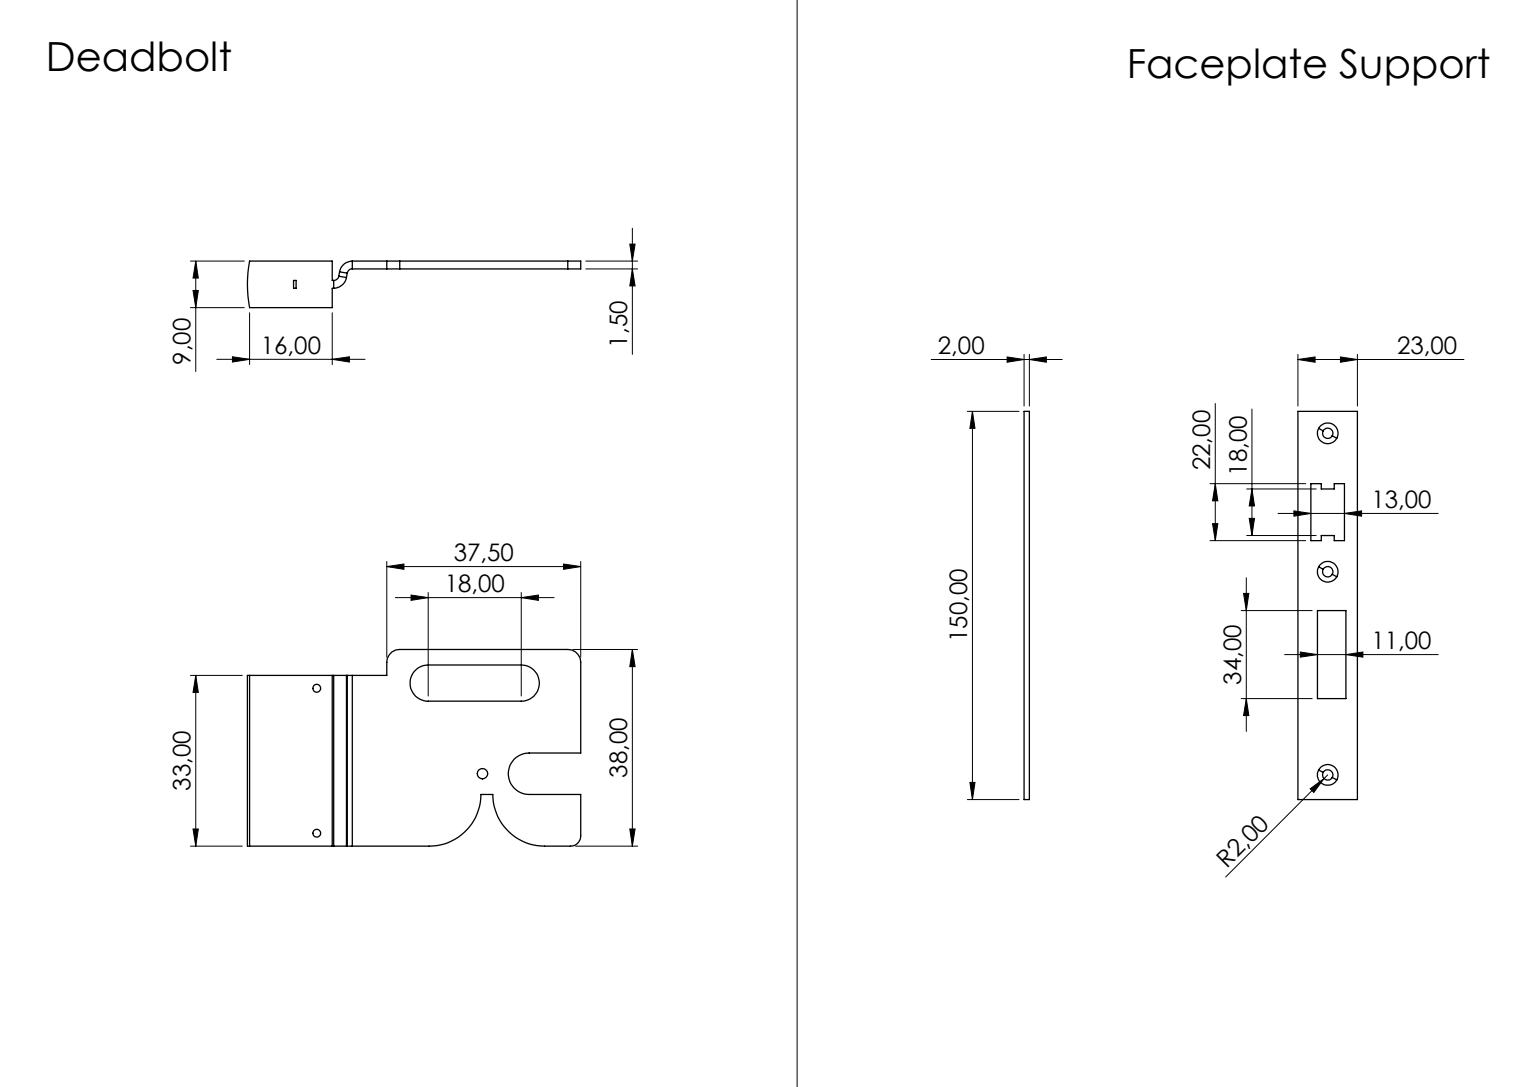
ISO-10303-21;
HEADER;
FILE_DESCRIPTION (('STEP AP214'),
    '1' );
FILE_NAME ('Deadbolt.step',
    '2026-10-06T13:23:30',
    ( '' ),
    ( '' ),
    'SwSTEP 2.0',
    'SolidWorks 2020',
    '' );
FILE_SCHEMA (( 'AUTOMOTIVE_DESIGN' ));
ENDSEC;

DATA;
#1=VERTEX_POINT ( 'NONE', #187 ) ;
#18=ORIENTED_EDGE ( 'NONE', *, *, #14112, .F. ) ;
#27=EDGE_LOOP ( 'NONE', ( #14113, #8328, #12180, #9090 ) ) ;
#42=DIRECTION ( 'NONE',  ( 0.000000000000000000, 1.000000000000000000, 0.000000000000000000 ) ) ;
#43=DIRECTION ( 'NONE',  ( 0.000000000000000000, 1.000000000000000000, 0.000000000000000000 ) ) ;
#46=CARTESIAN_POINT ( 'NONE',  ( -26.35824191589999899, -34.50000000000000000, -150.0657682190000060 ) ) ;
#49=DIRECTION ( 'NONE',  ( -2.507771768020000122E-12, -0.000000000000000000, 1.000000000000000000 ) ) ;
#77=AXIS2_PLACEMENT_3D ( 'NONE', #19282, #2992, #15716 ) ;
#116=MECHANICAL_DESIGN_GEOMETRIC_PRESENTATION_REPRESENTATION('',(#11103),#3517);
#123=CARTESIAN_POINT ( 'NONE',  ( 10.38320006080000013, -24.50000000000000000, -148.5552959529999839 ) ) ;
#126=DIRECTION ( 'NONE',  ( 0.000000000000000000, 0.000000000000000000, 1.000000000000000000 ) ) ;
#136=LINE ( 'NONE', #21434, #17431 ) ;
#139=CARTESIAN_POINT ( 'NONE',  ( -26.35824191589999899, -34.50000000000000000, -141.0657682190000060 ) ) ;
#140=CARTESIAN_POINT ( 'NONE',  ( -18.07392865170000107, -1.500000000000000000, -147.3157682190000060 ) ) ;
#154=VERTEX_POINT ( 'NONE', #4337 ) ;
#161=AXIS2_PLACEMENT_3D ( 'NONE', #17240, #17123, #840 ) ;
#163=DIRECTION ( 'NONE',  ( -2.808280234689999718E-18, 1.000000000000000000, 1.592654863519999645E-17 ) ) ;
#172=ADVANCED_FACE ( 'NONE', ( #21960 ), #4222, .F. ) ;
#175=CARTESIAN_POINT ( 'NONE',  ( -7.816799939239999162, -1.500000000000000000, -148.5552959529999839 ) ) ;
#176=DIRECTION ( 'NONE',  ( 2.507771768019999718E-12, 1.592654864069999939E-17, -1.000000000000000000 ) ) ;
#187=CARTESIAN_POINT ( 'NONE',  ( -20.60824191591068555, -32.00000000000000000, -141.9623572383543717 ) ) ;
#194=LINE ( 'NONE', #5434, #7982 ) ;
#197=CARTESIAN_POINT ( 'NONE',  ( -14.47770030809999930, -1.500000000000000000, -149.3052959529999839 ) ) ;
#200=ORIENTED_EDGE ( 'NONE', *, *, #6768, .F. ) ;
#209=STYLED_ITEM ( 'NONE', ( #19357 ), #4113 ) ;
#220=CARTESIAN_POINT ( 'NONE',  ( -16.93971969060000049, -1.500000000000000000, -147.9894163970000136 ) ) ;
#238=CARTESIAN_POINT ( 'NONE',  ( -7.816799939239999162, -0.2500000000010000334, -150.0552959529999839 ) ) ;
#241=CARTESIAN_POINT ( 'NONE',  ( -7.047250123649999587, -34.50000000000000000, -148.5552959529999839 ) ) ;
#246=VECTOR ( 'NONE', #23462, 1000.000000000000000 ) ;
#256=ADVANCED_FACE ( 'NONE', ( #12174 ), #12050, .F. ) ;
#264=ORIENTED_EDGE ( 'NONE', *, *, #15241, .F. ) ;
#270=CARTESIAN_POINT ( 'NONE',  ( 9.683200060760000838, -20.36785913719859664, -148.5552959529999839 ) ) ;
#273=DIRECTION ( 'NONE',  ( -1.000000000000000000, -3.994014902950000436E-29, 0.000000000000000000 ) ) ;
#279=EDGE_CURVE ( 'NONE', #18237, #3022, #18705, .T. ) ;
#334=FACE_OUTER_BOUND ( 'NONE', #6848, .T. ) ;
#338=AXIS2_PLACEMENT_3D ( 'NONE', #22132, #13076, #20347 ) ;
#351=DIRECTION ( 'NONE',  ( 0.000000000000000000, -1.000000000000000000, 0.000000000000000000 ) ) ;
#352=FACE_OUTER_BOUND ( 'NONE', #5067, .T. ) ;
#355=ORIENTED_EDGE ( 'NONE', *, *, #21836, .T. ) ;
#365=VECTOR ( 'NONE', #6982, 1000.000000000000000 ) ;
#371=CARTESIAN_POINT ( 'NONE',  ( 11.65767356897135443, -20.23976850042090092, -148.5552959529999839 ) ) ;
#382=DIRECTION ( 'NONE',  ( -1.000000000000000000, -3.994014902950000436E-29, 0.000000000000000000 ) ) ;
#388=CARTESIAN_POINT ( 'NONE',  ( 10.68320006080000084, -20.50000000000000000, -148.5552959529999839 ) ) ;
#393=EDGE_CURVE ( 'NONE', #3553, #18415, #4640, .T. ) ;
#394=ADVANCED_FACE ( 'NONE', ( #1724 ), #9053, .F. ) ;
#397=LINE ( 'NONE', #13222, #12316 ) ;
#402=VECTOR ( 'NONE', #1864, 1000.000000000000000 ) ;
#408=EDGE_LOOP ( 'NONE', ( #769, #22028, #13806, #15745 ) ) ;
#413=AXIS2_PLACEMENT_3D ( 'NONE', #5702, #16070, #23326 ) ;
#420=SURFACE_STYLE_FILL_AREA ( #21849 ) ;
#437=EDGE_CURVE ( 'NONE', #3022, #18237, #5403, .T. ) ;
#441=VECTOR ( 'NONE', #15364, 1000.000000000000000 ) ;
#443=AXIS2_PLACEMENT_3D ( 'NONE', #17861, #20351, #4284 ) ;
#458=CYLINDRICAL_SURFACE ( 'NONE', #11391, 10.00000000000000888 ) ;
#465=CARTESIAN_POINT ( 'NONE',  ( -22.10824191589999899, -32.00000000000000000, -146.2257682199999920 ) ) ;
#472=CARTESIAN_POINT ( 'NONE',  ( 22.68320006080000084, -34.50000000000000000, -148.5552959529999839 ) ) ;
#483=COLOUR_RGB ( '', 0.09019608, 0.27058824, 0.51372549) ;
#487=DIRECTION ( 'NONE',  ( -0.9848077530125620704, 4.409131086918041429E-28, -0.1736481776649230480 ) ) ;
#491=DIRECTION ( 'NONE',  ( 1.000000000000000000, 0.000000000000000000, 2.516505522483685870E-12 ) ) ;
#531=EDGE_CURVE ( 'NONE', #22008, #18104, #14787, .T. ) ;
#541=PRESENTATION_STYLE_ASSIGNMENT (( #8237 ) ) ;
#576=VERTEX_POINT ( 'NONE', #16915 ) ;
#601=DIRECTION ( 'NONE',  ( 0.000000000000000000, 0.000000000000000000, 1.000000000000000000 ) ) ;
#603=CARTESIAN_POINT ( 'NONE',  ( -22.10824191589623666, -4.196349540848737014, -146.3157682190018818 ) ) ;
#615=VECTOR ( 'NONE', #5815, 1000.000000000000000 ) ;
#629=ORIENTED_EDGE ( 'NONE', *, *, #11116, .F. ) ;
#640=ADVANCED_FACE ( 'NONE', ( #7633, #14906 ), #22163, .F. ) ;
#654=ORIENTED_EDGE ( 'NONE', *, *, #11108, .F. ) ;
#673=VECTOR ( 'NONE', #22152, 1000.000000000000000 ) ;
#676=EDGE_CURVE ( 'NONE', #3124, #23083, #5766, .T. ) ;
#679=EDGE_CURVE ( 'NONE', #5644, #19743, #22116, .T. ) ;
#680=VECTOR ( 'NONE', #351, 1000.000000000000000 ) ;
#691=CARTESIAN_POINT ( 'NONE',  ( -26.35824191589999899, -1.500000000000000000, -150.0657682190000060 ) ) ;
#702=EDGE_LOOP ( 'NONE', ( #22951, #2945, #10510, #19739 ) ) ;
#704=LINE ( 'NONE', #18543, #23404 ) ;
#723=AXIS2_PLACEMENT_3D ( 'NONE', #12821, #5462, #12706 ) ;
#733=CARTESIAN_POINT ( 'NONE',  ( -21.35824191589811605, -3.250000000000000000, -146.3157682190075093 ) ) ;
#740=CARTESIAN_POINT ( 'NONE',  ( -21.35824191589999899, -32.00000000000000000, -146.3157682190000060 ) ) ;
#768=EDGE_CURVE ( 'NONE', #11140, #3932, #17506, .T. ) ;
#769=ORIENTED_EDGE ( 'NONE', *, *, #15215, .F. ) ;
#789=AXIS2_PLACEMENT_3D ( 'NONE', #10567, #19991, #14634 ) ;
#793=DIRECTION ( 'NONE',  ( -2.507771768019999718E-12, -1.592654864069999939E-17, 1.000000000000000000 ) ) ;
#796=LINE ( 'NONE', #23004, #6121 ) ;
#797=ORIENTED_EDGE ( 'NONE', *, *, #13969, .F. ) ;
#814=CARTESIAN_POINT ( 'NONE',  ( 22.68320006080000084, -24.50000000000000000, -148.5552959529999839 ) ) ;
#827=ADVANCED_FACE ( 'NONE', ( #6913 ), #21441, .F. ) ;
#831=CARTESIAN_POINT ( 'NONE',  ( 11.53320006080000049, -24.50000000000000000, -148.5552959529999839 ) ) ;
#840=DIRECTION ( 'NONE',  ( 0.000000000000000000, -1.000000000000000000, -1.592654864069999939E-17 ) ) ;
#847=AXIS2_PLACEMENT_3D ( 'NONE', #18126, #23365, #1838 ) ;
#853=ORIENTED_EDGE ( 'NONE', *, *, #17082, .T. ) ;
#863=AXIS2_PLACEMENT_3D ( 'NONE', #7028, #8562, #12370 ) ;
#883=CARTESIAN_POINT ( 'NONE',  ( 19.68320006079999729, -24.50000000000000000, -149.3052959529999839 ) ) ;
#887=LINE ( 'NONE', #1123, #18501 ) ;
#892=ORIENTED_EDGE ( 'NONE', *, *, #13892, .T. ) ;
#909=DIRECTION ( 'NONE',  ( 0.000000000000000000, 0.000000000000000000, 1.000000000000000000 ) ) ;
#953=DIRECTION ( 'NONE',  ( 1.000000000000000000, 0.000000000000000000, 0.000000000000000000 ) ) ;
#958=FACE_BOUND ( 'NONE', #19822, .T. ) ;
#963=VERTEX_POINT ( 'NONE', #16860 ) ;
#973=CARTESIAN_POINT ( 'NONE',  ( -25.35824191589811960, -34.50000000000000000, -146.3157682190081346 ) ) ;
#978=EDGE_CURVE ( 'NONE', #17690, #8147, #22334, .T. ) ;
#1008=ORIENTED_EDGE ( 'NONE', *, *, #12992, .F. ) ;
#1043=CARTESIAN_POINT ( 'NONE',  ( -5.316799939240000938, 0.9999999999989999111, -150.0552959529999839 ) ) ;
#1044=CARTESIAN_POINT ( 'NONE',  ( -22.10824191589999899, -4.000000000000000000, -146.3157682190000060 ) ) ;
#1047=ORIENTED_EDGE ( 'NONE', *, *, #7201, .T. ) ;
#1050=CYLINDRICAL_SURFACE ( 'NONE', #8335, 0.7500000000000006661 ) ;
#1059=ORIENTED_EDGE ( 'NONE', *, *, #17973, .F. ) ;
#1060=DIRECTION ( 'NONE',  ( 1.000000000000000000, 1.387778780779999841E-17, 2.506439500389999993E-12 ) ) ;
#1061=FACE_OUTER_BOUND ( 'NONE', #22766, .T. ) ;
#1072=ORIENTED_EDGE ( 'NONE', *, *, #2514, .T. ) ;
#1073=CARTESIAN_POINT ( 'NONE',  ( -20.60824191589811605, -4.000000000000000000, -146.3157682190056335 ) ) ;
#1078=ADVANCED_FACE ( 'NONE', ( #18650 ), #15316, .F. ) ;
#1083=CARTESIAN_POINT ( 'NONE',  ( -25.35824191590000254, -18.00000000000000000, -144.8157682190000060 ) ) ;
#1105=CARTESIAN_POINT ( 'NONE',  ( 9.683200060759999062, -20.50000000000000000, -148.5552959529999839 ) ) ;
#1117=AXIS2_PLACEMENT_3D ( 'NONE', #140, #20122, #19888 ) ;
#1123=CARTESIAN_POINT ( 'NONE',  ( 29.68320006080000084, 0.9999999999989999111, -149.3052959529999839 ) ) ;
#1126=DIRECTION ( 'NONE',  ( 0.000000000000000000, 1.000000000000000000, 0.000000000000000000 ) ) ;
#1145=FACE_OUTER_BOUND ( 'NONE', #17569, .T. ) ;
#1151=EDGE_CURVE ( 'NONE', #8640, #1276, #4942, .T. ) ;
#1161=DIRECTION ( 'NONE',  ( 1.000000000000000000, 0.000000000000000000, 0.000000000000000000 ) ) ;
#1172=SURFACE_SIDE_STYLE ('',( #22576 ) ) ;
#1186=VERTEX_POINT ( 'NONE', #11465 ) ;
#1192=FACE_OUTER_BOUND ( 'NONE', #10960, .T. ) ;
#1194=VERTEX_POINT ( 'NONE', #4102 ) ;
#1202=CARTESIAN_POINT ( 'NONE',  ( -21.35824191589999899, -4.000000000000000000, -144.8157682190000060 ) ) ;
#1209=CIRCLE ( 'NONE', #14861, 2.500000000000000444 ) ;
#1213=DIRECTION ( 'NONE',  ( -1.000000000000000000, -3.994014904670000134E-29, 2.423380700840000070E-27 ) ) ;
#1214=CARTESIAN_POINT ( 'NONE',  ( -18.35824191589999899, -34.50000000000000000, -150.0657682190000060 ) ) ;
#1218=LINE ( 'NONE', #2868, #2873 ) ;
#1254=ORIENTED_EDGE ( 'NONE', *, *, #6417, .F. ) ;
#1259=EDGE_CURVE ( 'NONE', #3932, #4709, #8360, .T. ) ;
#1276=VERTEX_POINT ( 'NONE', #14824 ) ;
#1286=VERTEX_POINT ( 'NONE', #18625 ) ;
#1292=CARTESIAN_POINT ( 'NONE',  ( -21.74973190997081929, -3.330829822294064435, -146.3157682189990680 ) ) ;
#1326=FACE_OUTER_BOUND ( 'NONE', #18212, .T. ) ;
#1330=CARTESIAN_POINT ( 'NONE',  ( 19.68320006079999729, -16.50000000000000000, -150.0552959529999839 ) ) ;
#1340=DIRECTION ( 'NONE',  ( 0.000000000000000000, -1.000000000000000000, 0.000000000000000000 ) ) ;
#1352=AXIS2_PLACEMENT_3D ( 'NONE', #1566, #5353, #12601 ) ;
#1364=VERTEX_POINT ( 'NONE', #21003 ) ;
#1373=CARTESIAN_POINT ( 'NONE',  ( -20.60824191591068555, -4.000000000000000000, -141.9623572383543717 ) ) ;
#1402=CARTESIAN_POINT ( 'NONE',  ( -21.35824191589999899, -32.75000000000000000, -144.8157682190000060 ) ) ;
#1407=ADVANCED_FACE ( 'NONE', ( #12178 ), #12055, .F. ) ;
#1420=AXIS2_PLACEMENT_3D ( 'NONE', #23084, #17844, #15817 ) ;
#1426=CARTESIAN_POINT ( 'NONE',  ( 14.79224200840030257, -34.50000000000000000, -149.4708568728852356 ) ) ;
#1429=LINE ( 'NONE', #17483, #12868 ) ;
#1432=VECTOR ( 'NONE', #22263, 1000.000000000000000 ) ;
#1445=DIRECTION ( 'NONE',  ( 1.000000000000000000, 0.000000000000000000, 2.508689552389999873E-12 ) ) ;
#1468=LINE ( 'NONE', #22996, #9330 ) ;
#1493=CIRCLE ( 'NONE', #5705, 0.7500000000000006661 ) ;
#1494=CIRCLE ( 'NONE', #4516, 0.7500000000000006661 ) ;
#1509=AXIS2_PLACEMENT_3D ( 'NONE', #1202, #9968, #19028 ) ;
#1513=VERTEX_POINT ( 'NONE', #12648 ) ;
#1534=ORIENTED_EDGE ( 'NONE', *, *, #9605, .F. ) ;
#1552=FACE_OUTER_BOUND ( 'NONE', #10090, .T. ) ;
#1566=CARTESIAN_POINT ( 'NONE',  ( 18.18320006080000084, -3.000000000000000000, -148.5552959529999839 ) ) ;
#1573=LINE ( 'NONE', #16187, #18169 ) ;
#1576=ORIENTED_EDGE ( 'NONE', *, *, #7044, .F. ) ;
#1583=AXIS2_PLACEMENT_3D ( 'NONE', #11733, #4494, #6392 ) ;
#1587=CARTESIAN_POINT ( 'NONE',  ( 9.683200060759999062, -20.50000000000000000, -148.5552959529999839 ) ) ;
#1589=DIRECTION ( 'NONE',  ( -1.211690350419999855E-27, -2.765629237170000203E-27, 1.000000000000000000 ) ) ;
#1603=CARTESIAN_POINT ( 'NONE',  ( -18.35824191589999899, -1.500000000000000000, -146.3157682189915931 ) ) ;
#1604=FACE_OUTER_BOUND ( 'NONE', #8472, .T. ) ;
#1613=EDGE_CURVE ( 'NONE', #5042, #7140, #17473, .T. ) ;
#1617=AXIS2_PLACEMENT_3D ( 'NONE', #9994, #22985, #17152 ) ;
#1623=DIRECTION ( 'NONE',  ( 1.000000000000000000, 0.000000000000000000, 2.516505522483685870E-12 ) ) ;
#1631=UNCERTAINTY_MEASURE_WITH_UNIT (LENGTH_MEASURE( 1.000000000000000082E-05 ), #2207, 'distance_accuracy_value', 'NONE');
#1633=EDGE_LOOP ( 'NONE', ( #17440, #18528 ) ) ;
#1700=CARTESIAN_POINT ( 'NONE',  ( 10.55105919799721192, -21.49999999999999289, -148.5552959529999839 ) ) ;
#1724=FACE_OUTER_BOUND ( 'NONE', #16487, .T. ) ;
#1737=DIRECTION ( 'NONE',  ( 1.000000000000000000, 0.000000000000000000, 2.516505522483685870E-12 ) ) ;
#1742=EDGE_CURVE ( 'NONE', #3932, #15560, #19408, .T. ) ;
#1753=CARTESIAN_POINT ( 'NONE',  ( -21.35824191589999899, -32.00000000000000000, -141.0657682190000060 ) ) ;
#1761=AXIS2_PLACEMENT_3D ( 'NONE', #2604, #7594, #9833 ) ;
#1762=CARTESIAN_POINT ( 'NONE',  ( 10.68320006080000084, -20.50000000000000000, -148.5552959529999839 ) ) ;
#1765=ADVANCED_FACE ( 'NONE', ( #11049 ), #18207, .T. ) ;
#1771=DIRECTION ( 'NONE',  ( 3.994014902981375509E-29, -1.000000000000000000, 4.148443855750374987E-27 ) ) ;
#1792=FACE_BOUND ( 'NONE', #9087, .T. ) ;
#1801=CARTESIAN_POINT ( 'NONE',  ( 29.68320006080000084, -32.50000000000000000, -148.5552959529999839 ) ) ;
#1813=CARTESIAN_POINT ( 'NONE',  ( 9.810832519885522629, -21.00613386075831457, -148.5552959529999839 ) ) ;
#1835=EDGE_LOOP ( 'NONE', ( #19495, #20776, #3199, #14764 ) ) ;
#1837=EDGE_CURVE ( 'NONE', #576, #1513, #10267, .T. ) ;
#1838=DIRECTION ( 'NONE',  ( 1.000000000000000000, 0.000000000000000000, 2.507771768019999718E-12 ) ) ;
#1848=VECTOR ( 'NONE', #10158, 1000.000000000000000 ) ;
#1861=VERTEX_POINT ( 'NONE', #21673 ) ;
#1864=DIRECTION ( 'NONE',  ( 0.000000000000000000, 1.000000000000000000, 0.000000000000000000 ) ) ;
#1873=ORIENTED_EDGE ( 'NONE', *, *, #12997, .F. ) ;
#1880=LINE ( 'NONE', #197, #5897 ) ;
#1887=ORIENTED_EDGE ( 'NONE', *, *, #13153, .T. ) ;
#1911=DIRECTION ( 'NONE',  ( 0.000000000000000000, -1.000000000000000000, 0.000000000000000000 ) ) ;
#1932=CARTESIAN_POINT ( 'NONE',  ( 10.38320006080000013, -24.50000000000000000, -150.0552959529999839 ) ) ;
#1938=CARTESIAN_POINT ( 'NONE',  ( 10.42222808941079926, -21.47401663120255577, -148.5552959530000123 ) ) ;
#1950=ORIENTED_EDGE ( 'NONE', *, *, #3801, .F. ) ;
#1957=EDGE_CURVE ( 'NONE', #1276, #20629, #12257, .T. ) ;
#1963=EDGE_CURVE ( 'NONE', #10427, #4104, #7381, .T. ) ;
#1965=FACE_OUTER_BOUND ( 'NONE', #13295, .T. ) ;
#1968=AXIS2_PLACEMENT_3D ( 'NONE', #10420, #17698, #15908 ) ;
#1974=CARTESIAN_POINT ( 'NONE',  ( 19.68320006079999729, -20.50000000000000000, -150.0552959529999839 ) ) ;
#1988=VECTOR ( 'NONE', #12361, 1000.000000000000000 ) ;
#2011=ORIENTED_EDGE ( 'NONE', *, *, #13892, .F. ) ;
#2014=VERTEX_POINT ( 'NONE', #1932 ) ;
#2016=EDGE_CURVE ( 'NONE', #11959, #17690, #16433, .T. ) ;
#2018=ORIENTED_EDGE ( 'NONE', *, *, #12624, .T. ) ;
#2020=ORIENTED_EDGE ( 'NONE', *, *, #18687, .T. ) ;
#2040=DIRECTION ( 'NONE',  ( 1.000000000000000000, 0.000000000000000000, 0.000000000000000000 ) ) ;
#2072=VECTOR ( 'NONE', #16590, 1000.000000000000000 ) ;
#2093=ORIENTED_EDGE ( 'NONE', *, *, #19104, .T. ) ;
#2122=ORIENTED_EDGE ( 'NONE', *, *, #20027, .T. ) ;
#2129=EDGE_CURVE ( 'NONE', #17215, #6070, #6064, .T. ) ;
#2133=DIRECTION ( 'NONE',  ( 3.994014902821980611E-29, -1.000000000000000000, 4.148443855749775187E-27 ) ) ;
#2198=CARTESIAN_POINT ( 'NONE',  ( -21.35824191589999899, -32.00000000000000000, -144.8157682190000060 ) ) ;
#2207=( LENGTH_UNIT ( ) NAMED_UNIT ( * ) SI_UNIT ( .MILLI., .METRE. ) );
#2251=CIRCLE ( 'NONE', #10589, 1.000000000000000888 ) ;
#2252=CARTESIAN_POINT ( 'NONE',  ( 12.68320006080000084, -24.50000000000000000, -148.5552959529999839 ) ) ;
#2263=AXIS2_PLACEMENT_3D ( 'NONE', #16207, #18662, #23458 ) ;
#2269=AXIS2_PLACEMENT_3D ( 'NONE', #15309, #15537, #19221 ) ;
#2279=DIRECTION ( 'NONE',  ( -1.211690350419999855E-27, -2.765629237170000203E-27, 1.000000000000000000 ) ) ;
#2294=DIRECTION ( 'NONE',  ( -2.507771768019999718E-12, -1.592654864069999939E-17, 1.000000000000000000 ) ) ;
#2296=LINE ( 'NONE', #9166, #673 ) ;
#2317=FACE_OUTER_BOUND ( 'NONE', #19183, .T. ) ;
#2321=PLANE ( 'NONE',  #20385 ) ;
#2326=VECTOR ( 'NONE', #19118, 1000.000000000000000 ) ;
#2330=VERTEX_POINT ( 'NONE', #2615 ) ;
#2332=ADVANCED_FACE ( 'NONE', ( #9846 ), #19143, .F. ) ;
#2347=ORIENTED_EDGE ( 'NONE', *, *, #4982, .F. ) ;
#2368=LINE ( 'NONE', #22110, #18943 ) ;
#2369=CARTESIAN_POINT ( 'NONE',  ( -7.816799939239999162, 0.9999999999989999111, -148.5552959529999839 ) ) ;
#2373=AXIS2_PLACEMENT_3D ( 'NONE', #5090, #12334, #19611 ) ;
#2375=AXIS2_PLACEMENT_3D ( 'NONE', #5266, #23475, #273 ) ;
#2378=ORIENTED_EDGE ( 'NONE', *, *, #7878, .F. ) ;
#2384=CYLINDRICAL_SURFACE ( 'NONE', #1761, 2.500000000000002220 ) ;
#2393=VECTOR ( 'NONE', #601, 1000.000000000000000 ) ;
#2396=VERTEX_POINT ( 'NONE', #21617 ) ;
#2409=EDGE_CURVE ( 'NONE', #22806, #17118, #7206, .T. ) ;
#2442=LINE ( 'NONE', #9660, #21494 ) ;
#2444=DIRECTION ( 'NONE',  ( 0.000000000000000000, -1.000000000000000000, -1.592654864069999939E-17 ) ) ;
#2450=CARTESIAN_POINT ( 'NONE',  ( -22.10824191589999899, -4.000000000000000000, -146.3157682190000060 ) ) ;
#2466=CARTESIAN_POINT ( 'NONE',  ( -21.35824191589999899, -32.00000000000000000, -144.8157682190000060 ) ) ;
#2467=ORIENTED_EDGE ( 'NONE', *, *, #1151, .F. ) ;
#2486=EDGE_CURVE ( 'NONE', #6697, #2330, #18740, .T. ) ;
#2492=LINE ( 'NONE', #9367, #4851 ) ;
#2494=VERTEX_POINT ( 'NONE', #2450 ) ;
#2507=LINE ( 'NONE', #4393, #4653 ) ;
#2514=EDGE_CURVE ( 'NONE', #19622, #8290, #8123, .T. ) ;
#2517=DIRECTION ( 'NONE',  ( 1.000000000000000000, 0.000000000000000000, 2.516505522483685870E-12 ) ) ;
#2522=AXIS2_PLACEMENT_3D ( 'NONE', #14920, #19074, #18835 ) ;
#2534=ORIENTED_EDGE ( 'NONE', *, *, #14317, .T. ) ;
#2547=CARTESIAN_POINT ( 'NONE',  ( -34.35824191590000254, -18.00000000000000000, -150.0657682190000060 ) ) ;
#2552=CARTESIAN_POINT ( 'NONE',  ( -21.35824191589999899, -32.00000000000000000, -144.8157682190000060 ) ) ;
#2558=EDGE_CURVE ( 'NONE', #5708, #19622, #18777, .T. ) ;
#2563=ORIENTED_EDGE ( 'NONE', *, *, #18776, .T. ) ;
#2565=EDGE_CURVE ( 'NONE', #19064, #7036, #17058, .T. ) ;
#2588=CARTESIAN_POINT ( 'NONE',  ( -18.35824191589999899, -18.00000000000000000, -141.0657682190000060 ) ) ;
#2589=EDGE_CURVE ( 'NONE', #15557, #23525, #13250, .T. ) ;
#2594=DIRECTION ( 'NONE',  ( -0.9848077530125625145, 0.000000000000000000, -0.1736481776649201891 ) ) ;
#2600=CARTESIAN_POINT ( 'NONE',  ( -18.35824191589999899, -34.50000000000000000, -146.3157682190000060 ) ) ;
#2604=CARTESIAN_POINT ( 'NONE',  ( -18.07392865170000107, -18.00000000000000000, -147.3157682190000060 ) ) ;
#2608=ORIENTED_EDGE ( 'NONE', *, *, #16527, .T. ) ;
#2615=CARTESIAN_POINT ( 'NONE',  ( -14.47770030809999930, -1.500000000000000000, -148.5552959529999839 ) ) ;
#2621=DIRECTION ( 'NONE',  ( -1.211690350419999855E-27, -2.765629237170000203E-27, 1.000000000000000000 ) ) ;
#2627=FACE_OUTER_BOUND ( 'NONE', #22702, .T. ) ;
#2636=ORIENTED_EDGE ( 'NONE', *, *, #18562, .T. ) ;
#2649=EDGE_CURVE ( 'NONE', #1861, #6185, #21333, .T. ) ;
#2671=ORIENTED_EDGE ( 'NONE', *, *, #7178, .T. ) ;
#2676=ORIENTED_EDGE ( 'NONE', *, *, #13478, .F. ) ;
#2698=EDGE_CURVE ( 'NONE', #7704, #15634, #13963, .T. ) ;
#2713=CARTESIAN_POINT ( 'NONE',  ( -22.10824191589623311, -3.803650459151263874, -146.3157682190000344 ) ) ;
#2766=DIRECTION ( 'NONE',  ( -0.7071067811865474617, 0.7071067811865475727, 0.000000000000000000 ) ) ;
#2770=CARTESIAN_POINT ( 'NONE',  ( 0.3832000607639999834, -34.50000000000000000, -150.0552959529999839 ) ) ;
#2793=DIRECTION ( 'NONE',  ( 1.000000000000000000, 0.000000000000000000, 2.507771768019999718E-12 ) ) ;
#2820=( LENGTH_UNIT ( ) NAMED_UNIT ( * ) SI_UNIT ( .MILLI., .METRE. ) );
#2847=ORIENTED_EDGE ( 'NONE', *, *, #10102, .T. ) ;
#2861=ORIENTED_EDGE ( 'NONE', *, *, #11707, .F. ) ;
#2862=LINE ( 'NONE', #8439, #13539 ) ;
#2864=CARTESIAN_POINT ( 'NONE',  ( -20.60824191589999899, -32.00000000000000000, -150.0657682190000060 ) ) ;
#2868=CARTESIAN_POINT ( 'NONE',  ( -22.10824191589999899, -34.50000000000000000, -146.3157682190000060 ) ) ;
#2872=LINE ( 'NONE', #6434, #2995 ) ;
#2873=VECTOR ( 'NONE', #6427, 1000.000000000000000 ) ;
#2880=B_SPLINE_CURVE_WITH_KNOTS ( 'NONE', 3,
 ( #9732, #11287, #9621, #6297, #18691, #20594, #7729, #371, #22605, #16780 ),
 .UNSPECIFIED., .F., .F.,
 ( 4, 2, 2, 2, 4 ),
 ( 0.000000000000000000, 0.2500000000000000000, 0.5000000000000000000, 0.7500000000000000000, 1.000000000000000000 ),
 .UNSPECIFIED. ) ;
#2882=ORIENTED_EDGE ( 'NONE', *, *, #4143, .F. ) ;
#2895=DIRECTION ( 'NONE',  ( 0.000000000000000000, 0.000000000000000000, 1.000000000000000000 ) ) ;
#2928=CARTESIAN_POINT ( 'NONE',  ( 19.68320006079999729, -24.50000000000000000, -150.0552959529999839 ) ) ;
#2934=AXIS2_PLACEMENT_3D ( 'NONE', #2198, #7420, #5865 ) ;
#2936=EDGE_CURVE ( 'NONE', #6697, #963, #5850, .T. ) ;
#2942=CARTESIAN_POINT ( 'NONE',  ( -21.55459145674873866, -3.250000000000984102, -146.3157682189986133 ) ) ;
#2945=ORIENTED_EDGE ( 'NONE', *, *, #17078, .T. ) ;
#2957=EDGE_CURVE ( 'NONE', #1286, #6185, #20380, .T. ) ;
#2959=CARTESIAN_POINT ( 'NONE',  ( -18.07392865170000107, -18.00000000000000000, -147.3157682190000060 ) ) ;
#2976=PLANE ( 'NONE',  #18950 ) ;
#2992=DIRECTION ( 'NONE',  ( -2.507771768019999718E-12, -1.592654864069999939E-17, 1.000000000000000000 ) ) ;
#2995=VECTOR ( 'NONE', #22865, 1000.000000000000000 ) ;
#2999=VECTOR ( 'NONE', #17361, 1000.000000000000000 ) ;
#3019=AXIS2_PLACEMENT_3D ( 'NONE', #13523, #15082, #17336 ) ;
#3022=VERTEX_POINT ( 'NONE', #18586 ) ;
#3025=EDGE_CURVE ( 'NONE', #6070, #18790, #397, .T. ) ;
#3040=VERTEX_POINT ( 'NONE', #7750 ) ;
#3041=LINE ( 'NONE', #22661, #12557 ) ;
#3048=CARTESIAN_POINT ( 'NONE',  ( 10.38320006080000013, -24.50000000000000000, -149.3052959529999839 ) ) ;
#3067=SURFACE_STYLE_USAGE ( .BOTH. , #1172 ) ;
#3077=FACE_OUTER_BOUND ( 'NONE', #8007, .T. ) ;
#3078=ORIENTED_EDGE ( 'NONE', *, *, #9382, .T. ) ;
#3079=LINE ( 'NONE', #8166, #15110 ) ;
#3083=ORIENTED_EDGE ( 'NONE', *, *, #7044, .T. ) ;
#3094=CARTESIAN_POINT ( 'NONE',  ( -21.35824191589185972, -32.00000000000000000, -149.4708568729758724 ) ) ;
#3107=EDGE_CURVE ( 'NONE', #11140, #10546, #15835, .T. ) ;
#3114=AXIS2_PLACEMENT_3D ( 'NONE', #12481, #19993, #14399 ) ;
#3124=VERTEX_POINT ( 'NONE', #19059 ) ;
#3150=ADVANCED_FACE ( 'NONE', ( #4540 ), #4665, .F. ) ;
#3152=ORIENTED_EDGE ( 'NONE', *, *, #18916, .T. ) ;
#3173=VERTEX_POINT ( 'NONE', #2770 ) ;
#3186=DIRECTION ( 'NONE',  ( 1.000000000000000000, 0.000000000000000000, 2.507771768019999718E-12 ) ) ;
#3188=CARTESIAN_POINT ( 'NONE',  ( -22.10824191589999899, -4.000000000000000000, -141.0657682190000060 ) ) ;
#3199=ORIENTED_EDGE ( 'NONE', *, *, #20009, .T. ) ;
#3207=LINE ( 'NONE', #19264, #2999 ) ;
#3212=ORIENTED_EDGE ( 'NONE', *, *, #14784, .F. ) ;
#3222=CARTESIAN_POINT ( 'NONE',  ( 24.68320006080000084, -24.50000000000000000, -148.5552959529999839 ) ) ;
#3244=EDGE_LOOP ( 'NONE', ( #10415, #23135, #10407, #7914 ) ) ;
#3249=ORIENTED_EDGE ( 'NONE', *, *, #15929, .T. ) ;
#3251=EDGE_CURVE ( 'NONE', #20598, #12734, #9271, .T. ) ;
#3258=CARTESIAN_POINT ( 'NONE',  ( -21.35824191589999899, -32.00000000000000000, -150.0657682190000060 ) ) ;
#3277=EDGE_CURVE ( 'NONE', #154, #11758, #4731, .T. ) ;
#3309=VECTOR ( 'NONE', #16755, 1000.000000000000000 ) ;
#3315=DIRECTION ( 'NONE',  ( 0.000000000000000000, -4.148443855749999753E-27, -1.000000000000000000 ) ) ;
#3325=CARTESIAN_POINT ( 'NONE',  ( -5.316799939240000938, 3.500000000000000000, -149.3052959529999839 ) ) ;
#3327=DIRECTION ( 'NONE',  ( -1.211690350418039921E-27, -2.765629237168040089E-27, 1.000000000000000000 ) ) ;
#3332=CARTESIAN_POINT ( 'NONE',  ( -18.35824191589999899, -1.500000000000000000, -141.0657682190000060 ) ) ;
#3364=EDGE_CURVE ( 'NONE', #17304, #11140, #3467, .T. ) ;
#3375=CIRCLE ( 'NONE', #338, 0.7500000000000006661 ) ;
#3377=CARTESIAN_POINT ( 'NONE',  ( -16.79401156879999846, -18.00000000000000000, -148.8157682190000060 ) ) ;
#3422=ORIENTED_EDGE ( 'NONE', *, *, #17495, .F. ) ;
#3424=CYLINDRICAL_SURFACE ( 'NONE', #11993, 0.9999999999999950040 ) ;
#3444=LINE ( 'NONE', #16519, #19338 ) ;
#3450=DIRECTION ( 'NONE',  ( 0.000000000000000000, 0.000000000000000000, 1.000000000000000000 ) ) ;
#3459=LINE ( 'NONE', #12608, #1988 ) ;
#3467=LINE ( 'NONE', #12371, #4315 ) ;
#3473=EDGE_CURVE ( 'NONE', #17890, #2494, #11598, .T. ) ;
#3474=EDGE_CURVE ( 'NONE', #20840, #3553, #16707, .T. ) ;
#3489=ORIENTED_EDGE ( 'NONE', *, *, #531, .F. ) ;
#3500=AXIS2_PLACEMENT_3D ( 'NONE', #22901, #20758, #2793 ) ;
#3511=CARTESIAN_POINT ( 'NONE',  ( -21.35824191589999899, -4.000000000000000000, -144.8157682190000060 ) ) ;
#3517=( GEOMETRIC_REPRESENTATION_CONTEXT ( 3 ) GLOBAL_UNCERTAINTY_ASSIGNED_CONTEXT ( ( #20178 ) ) GLOBAL_UNIT_ASSIGNED_CONTEXT ( ( #15158, #6230, #13726 ) ) REPRESENTATION_CONTEXT ( 'NONE', 'WORKASPACE' ) );
#3543=CARTESIAN_POINT ( 'NONE',  ( -20.60824191589999899, -4.000000000000000000, -150.0657682190000060 ) ) ;
#3553=VERTEX_POINT ( 'NONE', #20819 ) ;
#3571=DIRECTION ( 'NONE',  ( -2.507771768019999718E-12, -1.592654864209999947E-17, 1.000000000000000000 ) ) ;
#3577=DIRECTION ( 'NONE',  ( 1.000000000000000000, 0.000000000000000000, 0.000000000000000000 ) ) ;
#3582=EDGE_CURVE ( 'NONE', #18490, #7197, #9850, .T. ) ;
#3587=CARTESIAN_POINT ( 'NONE',  ( -21.35824191589185972, -4.000000000000000000, -149.4708568729758724 ) ) ;
#3591=DIRECTION ( 'NONE',  ( -3.994014902950000436E-29, 1.000000000000000000, -4.148443855749999753E-27 ) ) ;
#3592=EDGE_CURVE ( 'NONE', #15090, #6658, #11014, .T. ) ;
#3603=ORIENTED_EDGE ( 'NONE', *, *, #18916, .F. ) ;
#3606=CARTESIAN_POINT ( 'NONE',  ( -12.87073128380000142, -1.500000000000000000, -149.4704070610000031 ) ) ;
#3620=DIRECTION ( 'NONE',  ( -3.994014902950000436E-29, 1.000000000000000000, -4.148443855749999753E-27 ) ) ;
#3657=VERTEX_POINT ( 'NONE', #1073 ) ;
#3695=EDGE_LOOP ( 'NONE', ( #4377, #20478, #21447, #5174 ) ) ;
#3702=CARTESIAN_POINT ( 'NONE',  ( 9.708726552585108749, -20.76023149958701453, -148.5552959529999839 ) ) ;
#3703=EDGE_CURVE ( 'NONE', #2014, #3173, #11377, .T. ) ;
#3719=PLANE ( 'NONE',  #12985 ) ;
#3720=EDGE_CURVE ( 'NONE', #1364, #12024, #17479, .T. ) ;
#3722=ORIENTED_EDGE ( 'NONE', *, *, #2957, .T. ) ;
#3724=PLANE ( 'NONE',  #18665 ) ;
#3729=VERTEX_POINT ( 'NONE', #23310 ) ;
#3767=DIRECTION ( 'NONE',  ( -2.508215857230000030E-12, 0.000000000000000000, 1.000000000000000000 ) ) ;
#3783=ORIENTED_EDGE ( 'NONE', *, *, #8938, .F. ) ;
#3801=EDGE_CURVE ( 'NONE', #17690, #3040, #15927, .T. ) ;
#3802=ORIENTED_EDGE ( 'NONE', *, *, #9650, .F. ) ;
#3804=FACE_OUTER_BOUND ( 'NONE', #15803, .T. ) ;
#3817=AXIS2_PLACEMENT_3D ( 'NONE', #9004, #12818, #18419 ) ;
#3828=VECTOR ( 'NONE', #5477, 1000.000000000000000 ) ;
#3868=EDGE_CURVE ( 'NONE', #15515, #5708, #21295, .T. ) ;
#3884=EDGE_CURVE ( 'NONE', #12276, #23083, #2368, .T. ) ;
#3897=ORIENTED_EDGE ( 'NONE', *, *, #22589, .T. ) ;
#3932=VERTEX_POINT ( 'NONE', #220 ) ;
#3933=DIRECTION ( 'NONE',  ( -0.1736481776649230480, 0.000000000000000000, 0.9848077530125620704 ) ) ;
#3935=ADVANCED_FACE ( 'NONE', ( #7919 ), #20090, .F. ) ;
#3947=CARTESIAN_POINT ( 'NONE',  ( -22.10824191589185972, -32.00000000000000000, -149.4708568729777483 ) ) ;
#3952=ORIENTED_EDGE ( 'NONE', *, *, #15367, .F. ) ;
#3953=LINE ( 'NONE', #11532, #13181 ) ;
#3979=PLANE ( 'NONE',  #21218 ) ;
#4008=EDGE_CURVE ( 'NONE', #2494, #9931, #13517, .T. ) ;
#4021=CARTESIAN_POINT ( 'NONE',  ( -20.60824191589999899, -4.000000000000000000, -146.2257682199999920 ) ) ;
#4028=CARTESIAN_POINT ( 'NONE',  ( 22.68320006080000084, -24.50000000000000000, -148.5552959529999839 ) ) ;
#4033=DIRECTION ( 'NONE',  ( 2.507771768020000122E-12, 0.000000000000000000, -1.000000000000000000 ) ) ;
#4050=DIRECTION ( 'NONE',  ( 2.507771768019999718E-12, 1.592654864209999947E-17, -1.000000000000000000 ) ) ;
#4052=ORIENTED_EDGE ( 'NONE', *, *, #22890, .T. ) ;
#4056=CIRCLE ( 'NONE', #7099, 0.7500000000000006661 ) ;
#4060=PLANE ( 'NONE',  #13489 ) ;
#4072=DIRECTION ( 'NONE',  ( 0.000000000000000000, 1.000000000000000000, 0.000000000000000000 ) ) ;
#4079=DIRECTION ( 'NONE',  ( 1.000000000000000000, 0.000000000000000000, 0.000000000000000000 ) ) ;
#4084=AXIS2_PLACEMENT_3D ( 'NONE', #15245, #11765, #15358 ) ;
#4096=ORIENTED_EDGE ( 'NONE', *, *, #20009, .F. ) ;
#4100=VERTEX_POINT ( 'NONE', #11964 ) ;
#4102=CARTESIAN_POINT ( 'NONE',  ( -7.816799939239999162, 0.9999999999989999111, -150.0552959529999839 ) ) ;
#4104=VERTEX_POINT ( 'NONE', #8273 ) ;
#4108=DIRECTION ( 'NONE',  ( -2.808280234689999718E-18, 1.000000000000000000, 1.592654863519999645E-17 ) ) ;
#4113=BREP_WITH_VOIDS ( 'NONE', #20590, ( #8159, #13114 ) );
#4138=CYLINDRICAL_SURFACE ( 'NONE', #17052, 2.499999999999999112 ) ;
#4143=EDGE_CURVE ( 'NONE', #10222, #3729, #18044, .T. ) ;
#4178=EDGE_LOOP ( 'NONE', ( #11998, #7794, #7453, #797 ) ) ;
#4185=DIRECTION ( 'NONE',  ( -1.000000000000000000, 0.000000000000000000, 0.000000000000000000 ) ) ;
#4215=CARTESIAN_POINT ( 'NONE',  ( -18.35824191589999899, -34.50000000000000000, -146.3157682190000060 ) ) ;
#4222=PLANE ( 'NONE',  #16412 ) ;
#4250=ORIENTED_EDGE ( 'NONE', *, *, #9936, .F. ) ;
#4278=ORIENTED_EDGE ( 'NONE', *, *, #9231, .F. ) ;
#4283=AXIS2_PLACEMENT_3D ( 'NONE', #1426, #21528, #8771 ) ;
#4284=DIRECTION ( 'NONE',  ( 1.000000000000000000, 0.000000000000000000, 0.000000000000000000 ) ) ;
#4297=EDGE_LOOP ( 'NONE', ( #19857, #13519, #13271, #15796 ) ) ;
#4299=FACE_OUTER_BOUND ( 'NONE', #1835, .T. ) ;
#4315=VECTOR ( 'NONE', #19648, 1000.000000000000227 ) ;
#4327=CARTESIAN_POINT ( 'NONE',  ( 0.1832000607640000001, 0.4999999999990000776, -149.3052959529999839 ) ) ;
#4333=EDGE_CURVE ( 'NONE', #15560, #8780, #11225, .T. ) ;
#4337=CARTESIAN_POINT ( 'NONE',  ( -22.10824191589186327, -4.000000000000000000, -149.4708568729739966 ) ) ;
#4354=LINE ( 'NONE', #11706, #1848 ) ;
#4368=ORIENTED_EDGE ( 'NONE', *, *, #22047, .T. ) ;
#4372=ORIENTED_EDGE ( 'NONE', *, *, #9872, .F. ) ;
#4377=ORIENTED_EDGE ( 'NONE', *, *, #6622, .T. ) ;
#4384=ORIENTED_EDGE ( 'NONE', *, *, #18993, .F. ) ;
#4393=CARTESIAN_POINT ( 'NONE',  ( -17.01442029460000072, -1.500000000000000000, -147.5657682190000060 ) ) ;
#4398=DIRECTION ( 'NONE',  ( -1.211690350419999855E-27, -2.765629237169980113E-27, 1.000000000000000000 ) ) ;
#4415=CARTESIAN_POINT ( 'NONE',  ( 10.68320006080000084, -19.50000000000000000, -148.5552959529999839 ) ) ;
#4419=DIRECTION ( 'NONE',  ( -1.211690350419999855E-27, -2.765629237170000203E-27, 1.000000000000000000 ) ) ;
#4421=ORIENTED_EDGE ( 'NONE', *, *, #22935, .F. ) ;
#4428=FACE_OUTER_BOUND ( 'NONE', #13600, .T. ) ;
#4451=CARTESIAN_POINT ( 'NONE',  ( 10.68320006080000084, -19.50000000000000000, -149.3052959529999839 ) ) ;
#4492=ORIENTED_EDGE ( 'NONE', *, *, #6187, .F. ) ;
#4494=DIRECTION ( 'NONE',  ( -2.507771768019999718E-12, -1.592654864069999939E-17, 1.000000000000000000 ) ) ;
#4495=EDGE_LOOP ( 'NONE', ( #2676, #13552, #21698, #22176 ) ) ;
#4516=AXIS2_PLACEMENT_3D ( 'NONE', #13322, #7957, #7610 ) ;
#4527=CARTESIAN_POINT ( 'NONE',  ( -20.96675192182589953, -3.330829822291216047, -146.3157682189990396 ) ) ;
#4540=FACE_OUTER_BOUND ( 'NONE', #16138, .T. ) ;
#4560=PLANE ( 'NONE',  #16687 ) ;
#4562=DIRECTION ( 'NONE',  ( 0.000000000000000000, 0.000000000000000000, 1.000000000000000000 ) ) ;
#4575=DIRECTION ( 'NONE',  ( 3.994014902950000436E-29, -1.000000000000000000, 4.148443855749999753E-27 ) ) ;
#4581=AXIS2_PLACEMENT_3D ( 'NONE', #10494, #3620, #6829 ) ;
#4590=CARTESIAN_POINT ( 'NONE',  ( 0.000000000000000000, 0.000000000000000000, 0.000000000000000000 ) ) ;
#4600=EDGE_CURVE ( 'NONE', #15711, #1194, #22364, .T. ) ;
#4605=LINE ( 'NONE', #20671, #8067 ) ;
#4623=DIRECTION ( 'NONE',  ( 0.000000000000000000, -1.000000000000000000, -2.765629237170000203E-27 ) ) ;
#4630=ORIENTED_EDGE ( 'NONE', *, *, #2936, .T. ) ;
#4640=CIRCLE ( 'NONE', #11074, 0.7500000000000006661 ) ;
#4642=DIRECTION ( 'NONE',  ( -2.507771768019999718E-12, -1.592654864069999939E-17, 1.000000000000000000 ) ) ;
#4653=VECTOR ( 'NONE', #22140, 1000.000000000000227 ) ;
#4665=PLANE ( 'NONE',  #7007 ) ;
#4692=CARTESIAN_POINT ( 'NONE',  ( -21.71608528380000180, -1.500000000000000000, -146.3157682190000060 ) ) ;
#4696=ORIENTED_EDGE ( 'NONE', *, *, #21770, .F. ) ;
#4701=ADVANCED_FACE ( 'NONE', ( #2627 ), #22606, .T. ) ;
#4704=CARTESIAN_POINT ( 'NONE',  ( 29.68320006080000084, -16.50000000000000000, -150.0552959529999839 ) ) ;
#4709=VERTEX_POINT ( 'NONE', #6299 ) ;
#4715=ORIENTED_EDGE ( 'NONE', *, *, #10137, .T. ) ;
#4731=CIRCLE ( 'NONE', #21461, 0.7500000000000006661 ) ;
#4734=CARTESIAN_POINT ( 'NONE',  ( 18.18320006080000084, -3.000000000000000000, -150.0552959529999839 ) ) ;
#4738=DIRECTION ( 'NONE',  ( -0.6427876096862108479, 0.000000000000000000, -0.7660444431192537929 ) ) ;
#4770=FACE_OUTER_BOUND ( 'NONE', #22126, .T. ) ;
#4772=VECTOR ( 'NONE', #6547, 1000.000000000000000 ) ;
#4789=CIRCLE ( 'NONE', #2522, 0.7500000000000006661 ) ;
#4814=DIRECTION ( 'NONE',  ( -2.507771768019999718E-12, -1.592654864069999939E-17, 1.000000000000000000 ) ) ;
#4829=EDGE_LOOP ( 'NONE', ( #8714, #3802, #14735, #6395 ) ) ;
#4833=ORIENTED_EDGE ( 'NONE', *, *, #19853, .T. ) ;
#4838=FACE_OUTER_BOUND ( 'NONE', #20075, .T. ) ;
#4841=FACE_OUTER_BOUND ( 'NONE', #21996, .T. ) ;
#4842=EDGE_LOOP ( 'NONE', ( #20125, #22858, #14646, #16712 ) ) ;
#4850=DIRECTION ( 'NONE',  ( 0.000000000000000000, 0.000000000000000000, 1.000000000000000000 ) ) ;
#4851=VECTOR ( 'NONE', #16760, 1000.000000000000000 ) ;
#4880=CARTESIAN_POINT ( 'NONE',  ( -22.10824191589999899, -4.000000000000000000, -145.5657682190000060 ) ) ;
#4898=EDGE_CURVE ( 'NONE', #6741, #11959, #5656, .T. ) ;
#4910=DIRECTION ( 'NONE',  ( 1.000000000000000000, 0.000000000000000000, 2.507771768019999718E-12 ) ) ;
#4942=CIRCLE ( 'NONE', #18630, 0.7500000000000006661 ) ;
#4952=EDGE_CURVE ( 'NONE', #4709, #22352, #16057, .T. ) ;
#4963=VECTOR ( 'NONE', #6909, 1000.000000000000000 ) ;
#4969=CARTESIAN_POINT ( 'NONE',  ( -17.23482902069999767, -18.00000000000000000, -144.8157682190000060 ) ) ;
#4982=EDGE_CURVE ( 'NONE', #5391, #576, #3444, .T. ) ;
#5018=DIRECTION ( 'NONE',  ( -1.000000000000000000, -3.994014902950000436E-29, 0.000000000000000000 ) ) ;
#5023=ORIENTED_EDGE ( 'NONE', *, *, #679, .F. ) ;
#5025=AXIS2_PLACEMENT_3D ( 'NONE', #4590, #17084, #1161 ) ;
#5028=AXIS2_PLACEMENT_3D ( 'NONE', #20089, #7692, #9245 ) ;
#5042=VERTEX_POINT ( 'NONE', #17102 ) ;
#5047=( GEOMETRIC_REPRESENTATION_CONTEXT ( 3 ) GLOBAL_UNCERTAINTY_ASSIGNED_CONTEXT ( ( #1631 ) ) GLOBAL_UNIT_ASSIGNED_CONTEXT ( ( #2207, #22188, #9311 ) ) REPRESENTATION_CONTEXT ( 'NONE', 'WORKASPACE' ) );
#5054=PLANE ( 'NONE',  #8381 ) ;
#5055=EDGE_CURVE ( 'NONE', #1186, #10902, #22461, .T. ) ;
#5060=EDGE_CURVE ( 'NONE', #1276, #8640, #22011, .T. ) ;
#5061=DIRECTION ( 'NONE',  ( 2.507554887169999917E-12, 0.000000000000000000, -1.000000000000000000 ) ) ;
#5067=EDGE_LOOP ( 'NONE', ( #7161, #6503, #20402, #13366 ) ) ;
#5082=DIRECTION ( 'NONE',  ( -2.507771768019999718E-12, -1.592654864069999939E-17, 1.000000000000000000 ) ) ;
#5084=CARTESIAN_POINT ( 'NONE',  ( -21.35824191589185972, -4.000000000000000000, -149.4708568729758724 ) ) ;
#5087=CARTESIAN_POINT ( 'NONE',  ( -14.47770030809999930, -34.50000000000000000, -149.3052959529999839 ) ) ;
#5090=CARTESIAN_POINT ( 'NONE',  ( 19.68320006079999729, -20.50000000000000000, -148.5552959529999839 ) ) ;
#5105=VECTOR ( 'NONE', #8484, 1000.000000000000000 ) ;
#5114=LINE ( 'NONE', #10565, #11202 ) ;
#5117=DIRECTION ( 'NONE',  ( 1.000000000000000000, 0.000000000000000000, 2.504935852220000146E-12 ) ) ;
#5150=ORIENTED_EDGE ( 'NONE', *, *, #23485, .F. ) ;
#5155=ORIENTED_EDGE ( 'NONE', *, *, #13911, .T. ) ;
#5157=ADVANCED_FACE ( 'NONE', ( #13291 ), #4138, .T. ) ;
#5172=ORIENTED_EDGE ( 'NONE', *, *, #7232, .F. ) ;
#5174=ORIENTED_EDGE ( 'NONE', *, *, #5620, .F. ) ;
#5199=AXIS2_PLACEMENT_3D ( 'NONE', #18505, #4108, #22314 ) ;
#5204=AXIS2_PLACEMENT_3D ( 'NONE', #7588, #14627, #15408 ) ;
#5223=CARTESIAN_POINT ( 'NONE',  ( -20.70396626025547349, -4.379374642480768465, -146.3157682190058893 ) ) ;
#5245=DIRECTION ( 'NONE',  ( 2.506794771760000178E-12, 0.000000000000000000, -1.000000000000000000 ) ) ;
#5247=EDGE_LOOP ( 'NONE', ( #18873, #12800, #10794, #13305, #9427, #9623, #12391, #264 ) ) ;
#5249=PLANE ( 'NONE',  #10604 ) ;
#5266=CARTESIAN_POINT ( 'NONE',  ( -17.08727435560000174, -1.500000000000000000, -147.1525923079999814 ) ) ;
#5273=DIRECTION ( 'NONE',  ( 2.507771768019999718E-12, 1.592654864069999939E-17, -1.000000000000000000 ) ) ;
#5291=VECTOR ( 'NONE', #2895, 1000.000000000000000 ) ;
#5329=EDGE_LOOP ( 'NONE', ( #17673, #19947, #5172, #5455, #22802, #18163, #5335, #629, #6248, #5793, #13808, #4278, #4421, #11355, #853, #17481, #20909 ) ) ;
#5335=ORIENTED_EDGE ( 'NONE', *, *, #8346, .F. ) ;
#5346=PLANE ( 'NONE',  #723 ) ;
#5349=ORIENTED_EDGE ( 'NONE', *, *, #17458, .T. ) ;
#5353=DIRECTION ( 'NONE',  ( -1.211690350419999855E-27, -2.765629237170000203E-27, 1.000000000000000000 ) ) ;
#5386=AXIS2_PLACEMENT_3D ( 'NONE', #740, #20373, #18464 ) ;
#5390=CARTESIAN_POINT ( 'NONE',  ( -21.35824191589999899, -32.00000000000000000, -144.8157682190000060 ) ) ;
#5391=VERTEX_POINT ( 'NONE', #9325 ) ;
#5403=CIRCLE ( 'NONE', #10311, 0.7500000000000006661 ) ;
#5404=EDGE_LOOP ( 'NONE', ( #14480, #6053, #2018, #11835 ) ) ;
#5433=EDGE_LOOP ( 'NONE', ( #14124, #12310 ) ) ;
#5434=CARTESIAN_POINT ( 'NONE',  ( -7.047250123649999587, -34.50000000000000000, -150.0552959529999839 ) ) ;
#5445=LINE ( 'NONE', #21516, #17024 ) ;
#5453=ORIENTED_EDGE ( 'NONE', *, *, #2409, .F. ) ;
#5455=ORIENTED_EDGE ( 'NONE', *, *, #19894, .F. ) ;
#5457=PLANE ( 'NONE',  #20241 ) ;
#5458=ORIENTED_EDGE ( 'NONE', *, *, #22202, .F. ) ;
#5462=DIRECTION ( 'NONE',  ( -1.000000000000000000, -2.808280234649999694E-18, -2.507771768019999718E-12 ) ) ;
#5477=DIRECTION ( 'NONE',  ( 0.000000000000000000, -1.000000000000000000, 0.000000000000000000 ) ) ;
#5503=LINE ( 'NONE', #16335, #6761 ) ;
#5581=VECTOR ( 'NONE', #17669, 1000.000000000000000 ) ;
#5599=DIRECTION ( 'NONE',  ( 1.000000000000000000, 0.000000000000000000, 0.000000000000000000 ) ) ;
#5606=CARTESIAN_POINT ( 'NONE',  ( -21.71608528380000180, -34.50000000000000000, -144.8157682190000060 ) ) ;
#5607=CARTESIAN_POINT ( 'NONE',  ( 29.68320006080000084, -16.50000000000000000, -148.5552959529999839 ) ) ;
#5614=LINE ( 'NONE', #12866, #14362 ) ;
#5620=EDGE_CURVE ( 'NONE', #23525, #9016, #18831, .T. ) ;
#5644=VERTEX_POINT ( 'NONE', #8224 ) ;
#5656=CIRCLE ( 'NONE', #14396, 25.00000000000000000 ) ;
#5665=ORIENTED_EDGE ( 'NONE', *, *, #1742, .T. ) ;
#5670=EDGE_LOOP ( 'NONE', ( #21435, #2534, #10146, #11717 ) ) ;
#5674=ORIENTED_EDGE ( 'NONE', *, *, #7232, .T. ) ;
#5682=DIRECTION ( 'NONE',  ( -3.994014902950000436E-29, 1.000000000000000000, -4.148443855749999753E-27 ) ) ;
#5685=AXIS2_PLACEMENT_3D ( 'NONE', #6054, #22591, #4623 ) ;
#5688=DIRECTION ( 'NONE',  ( 0.000000000000000000, 1.000000000000000000, 0.000000000000000000 ) ) ;
#5702=CARTESIAN_POINT ( 'NONE',  ( 18.18320006080000084, -3.000000000000000000, -148.5552959529999839 ) ) ;
#5705=AXIS2_PLACEMENT_3D ( 'NONE', #14214, #19684, #1623 ) ;
#5708=VERTEX_POINT ( 'NONE', #22639 ) ;
#5716=DIRECTION ( 'NONE',  ( 1.000000000000000000, 0.000000000000000000, 0.000000000000000000 ) ) ;
#5730=DIRECTION ( 'NONE',  ( 2.507771768020000122E-12, 0.000000000000000000, -1.000000000000000000 ) ) ;
#5735=CARTESIAN_POINT ( 'NONE',  ( 9.882979739358319193, -19.88614550847407259, -148.5552959529999839 ) ) ;
#5736=EDGE_CURVE ( 'NONE', #1194, #11089, #18726, .T. ) ;
#5740=ORIENTED_EDGE ( 'NONE', *, *, #1259, .T. ) ;
#5766=CIRCLE ( 'NONE', #8796, 2.000000000000001776 ) ;
#5778=PLANE ( 'NONE',  #5199 ) ;
#5782=LINE ( 'NONE', #13041, #7269 ) ;
#5790=CARTESIAN_POINT ( 'NONE',  ( -34.35824191590000254, -1.500000000000000000, -150.0657682190000060 ) ) ;
#5793=ORIENTED_EDGE ( 'NONE', *, *, #6622, .F. ) ;
#5810=PLANE ( 'NONE',  #10912 ) ;
#5815=DIRECTION ( 'NONE',  ( -1.000000000000000000, 0.000000000000000000, 0.000000000000000000 ) ) ;
#5825=CYLINDRICAL_SURFACE ( 'NONE', #18334, 0.7500000000000016653 ) ;
#5847=VECTOR ( 'NONE', #1340, 1000.000000000000000 ) ;
#5849=CARTESIAN_POINT ( 'NONE',  ( -21.71608528419999828, -34.50000000000000000, -144.8157682190000060 ) ) ;
#5850=LINE ( 'NONE', #6212, #10778 ) ;
#5855=ADVANCED_FACE ( 'NONE', ( #16088 ), #5249, .T. ) ;
#5862=LINE ( 'NONE', #17168, #5919 ) ;
#5865=DIRECTION ( 'NONE',  ( 1.000000000000000000, 0.000000000000000000, 2.516505522483685870E-12 ) ) ;
#5878=DIRECTION ( 'NONE',  ( 0.000000000000000000, 0.000000000000000000, 1.000000000000000000 ) ) ;
#5882=EDGE_CURVE ( 'NONE', #7389, #7704, #6570, .T. ) ;
#5890=FACE_OUTER_BOUND ( 'NONE', #5247, .T. ) ;
#5897=VECTOR ( 'NONE', #9104, 1000.000000000000000 ) ;
#5919=VECTOR ( 'NONE', #16930, 1000.000000000000000 ) ;
#5928=LINE ( 'NONE', #22473, #615 ) ;
#5941=DIRECTION ( 'NONE',  ( -2.510584333019999972E-12, 0.000000000000000000, 1.000000000000000000 ) ) ;
#5955=ORIENTED_EDGE ( 'NONE', *, *, #6555, .T. ) ;
#5963=EDGE_CURVE ( 'NONE', #8780, #19806, #14969, .T. ) ;
#5965=VECTOR ( 'NONE', #18837, 1000.000000000000000 ) ;
#5971=ORIENTED_EDGE ( 'NONE', *, *, #21770, .T. ) ;
#5989=ORIENTED_EDGE ( 'NONE', *, *, #437, .T. ) ;
#5991=ORIENTED_EDGE ( 'NONE', *, *, #19570, .T. ) ;
#6006=ADVANCED_FACE ( 'NONE', ( #11381 ), #7816, .F. ) ;
#6023=ORIENTED_EDGE ( 'NONE', *, *, #3107, .T. ) ;
#6028=FACE_OUTER_BOUND ( 'NONE', #3244, .T. ) ;
#6053=ORIENTED_EDGE ( 'NONE', *, *, #2936, .F. ) ;
#6054=CARTESIAN_POINT ( 'NONE',  ( 10.93320006080000084, -15.50000000000000000, -148.5552959529999839 ) ) ;
#6064=LINE ( 'NONE', #13315, #7981 ) ;
#6070=VERTEX_POINT ( 'NONE', #18886 ) ;
#6081=VECTOR ( 'NONE', #21532, 1000.000000000000000 ) ;
#6083=DIRECTION ( 'NONE',  ( 2.507771768019999718E-12, 1.592654864069999939E-17, -1.000000000000000000 ) ) ;
#6104=ORIENTED_EDGE ( 'NONE', *, *, #8207, .F. ) ;
#6106=DIRECTION ( 'NONE',  ( -2.507771768019999718E-12, -1.592654864209999947E-17, 1.000000000000000000 ) ) ;
#6121=VECTOR ( 'NONE', #20773, 1000.000000000000227 ) ;
#6122=CLOSED_SHELL ( 'NONE', ( #22066, #1078, #20319, #14625, #22671, #6006 ) ) ;
#6135=DIRECTION ( 'NONE',  ( 0.7071067811865499042, -0.7071067811865451302, 1.776356839400251071E-12 ) ) ;
#6137=VECTOR ( 'NONE', #11195, 1000.000000000000000 ) ;
#6150=DIRECTION ( 'NONE',  ( -1.387778780781445676E-15, 1.000000000000000000, 0.000000000000000000 ) ) ;
#6166=DIRECTION ( 'NONE',  ( -1.000000000000000000, 0.000000000000000000, 0.000000000000000000 ) ) ;
#6169=LINE ( 'NONE', #11393, #19766 ) ;
#6183=ADVANCED_FACE ( 'NONE', ( #17337 ), #1050, .F. ) ;
#6185=VERTEX_POINT ( 'NONE', #12441 ) ;
#6187=EDGE_CURVE ( 'NONE', #18415, #6658, #18167, .T. ) ;
#6188=VERTEX_POINT ( 'NONE', #12213 ) ;
#6207=DIRECTION ( 'NONE',  ( 1.000000000000000000, 0.000000000000000000, 0.000000000000000000 ) ) ;
#6212=CARTESIAN_POINT ( 'NONE',  ( -7.816799939239999162, -1.500000000000000000, -149.3052959529999839 ) ) ;
#6213=ORIENTED_EDGE ( 'NONE', *, *, #19853, .F. ) ;
#6214=CARTESIAN_POINT ( 'NONE',  ( -22.10824191589999899, -4.000000000000000000, -146.2257682199999920 ) ) ;
#6215=DIRECTION ( 'NONE',  ( 0.000000000000000000, 0.000000000000000000, 1.000000000000000000 ) ) ;
#6230=( NAMED_UNIT ( * ) PLANE_ANGLE_UNIT ( ) SI_UNIT ( $, .RADIAN. ) );
#6231=ADVANCED_FACE ( 'NONE', ( #7101 ), #10769, .F. ) ;
#6241=DIRECTION ( 'NONE',  ( -1.000000000000000000, 0.000000000000000000, 0.000000000000000000 ) ) ;
#6248=ORIENTED_EDGE ( 'NONE', *, *, #14188, .F. ) ;
#6276=ORIENTED_EDGE ( 'NONE', *, *, #18687, .F. ) ;
#6277=LINE ( 'NONE', #831, #11305 ) ;
#6289=ORIENTED_EDGE ( 'NONE', *, *, #15028, .F. ) ;
#6294=VECTOR ( 'NONE', #909, 1000.000000000000000 ) ;
#6297=CARTESIAN_POINT ( 'NONE',  ( 11.18859344972421788, -19.62717558213227420, -148.5552959529999555 ) ) ;
#6299=CARTESIAN_POINT ( 'NONE',  ( -14.47770030809999930, -1.500000000000000000, -150.0552959529999839 ) ) ;
#6303=ADVANCED_FACE ( 'NONE', ( #10654 ), #14597, .T. ) ;
#6309=CIRCLE ( 'NONE', #16569, 0.7500000000000006661 ) ;
#6315=CARTESIAN_POINT ( 'NONE',  ( 0.3832000607639999834, -24.50000000000000000, -148.5552959529999839 ) ) ;
#6319=CARTESIAN_POINT ( 'NONE',  ( -15.46250806109999942, -18.00000000000000000, -147.7289441310000200 ) ) ;
#6341=CIRCLE ( 'NONE', #12803, 4.000000000000000000 ) ;
#6343=ADVANCED_FACE ( 'NONE', ( #5890, #14705 ), #5778, .T. ) ;
#6365=CYLINDRICAL_SURFACE ( 'NONE', #13217, 0.7499999999999997780 ) ;
#6392=DIRECTION ( 'NONE',  ( 1.000000000000000000, 0.000000000000000000, 2.507771768019999718E-12 ) ) ;
#6395=ORIENTED_EDGE ( 'NONE', *, *, #21298, .T. ) ;
#6407=DIRECTION ( 'NONE',  ( -2.507771768022264771E-12, -1.592655090489709912E-17, 1.000000000000000000 ) ) ;
#6410=VECTOR ( 'NONE', #21522, 1000.000000000000000 ) ;
#6417=EDGE_CURVE ( 'NONE', #17085, #7870, #7787, .T. ) ;
#6423=CARTESIAN_POINT ( 'NONE',  ( -11.14725012360000100, -1.500000000000000000, -150.0552959529999839 ) ) ;
#6425=ORIENTED_EDGE ( 'NONE', *, *, #19681, .F. ) ;
#6427=DIRECTION ( 'NONE',  ( 1.000000000000000000, 0.000000000000000000, 2.504899991129999675E-12 ) ) ;
#6433=AXIS2_PLACEMENT_3D ( 'NONE', #4028, #11151, #18424 ) ;
#6434=CARTESIAN_POINT ( 'NONE',  ( -21.35824191589999899, -3.250000000000000000, -145.5657682190000060 ) ) ;
#6441=AXIS2_PLACEMENT_3D ( 'NONE', #4969, #19492, #3186 ) ;
#6455=DIRECTION ( 'NONE',  ( 0.000000000000000000, 0.000000000000000000, 1.000000000000000000 ) ) ;
#6469=CIRCLE ( 'NONE', #21999, 1.000000000000000888 ) ;
#6494=ORIENTED_EDGE ( 'NONE', *, *, #1742, .F. ) ;
#6502=ADVANCED_FACE ( 'NONE', ( #19815 ), #12304, .F. ) ;
#6503=ORIENTED_EDGE ( 'NONE', *, *, #21298, .F. ) ;
#6514=CIRCLE ( 'NONE', #3114, 2.000000000000001776 ) ;
#6520=ORIENTED_EDGE ( 'NONE', *, *, #3720, .T. ) ;
#6532=ORIENTED_EDGE ( 'NONE', *, *, #3582, .F. ) ;
#6547=DIRECTION ( 'NONE',  ( -1.000000000000000000, 0.000000000000000000, -2.508689552389999873E-12 ) ) ;
#6555=EDGE_CURVE ( 'NONE', #8640, #1, #14332, .T. ) ;
#6570=LINE ( 'NONE', #10472, #14417 ) ;
#6571=ORIENTED_EDGE ( 'NONE', *, *, #7497, .F. ) ;
#6583=ORIENTED_EDGE ( 'NONE', *, *, #17066, .T. ) ;
#6617=DIRECTION ( 'NONE',  ( -1.211690350419999855E-27, -2.765629237170000203E-27, 1.000000000000000000 ) ) ;
#6622=EDGE_CURVE ( 'NONE', #23525, #20598, #6341, .T. ) ;
#6646=ORIENTED_EDGE ( 'NONE', *, *, #7785, .F. ) ;
#6658=VERTEX_POINT ( 'NONE', #16468 ) ;
#6663=LINE ( 'NONE', #13927, #17161 ) ;
#6666=AXIS2_PLACEMENT_3D ( 'NONE', #15300, #793, #11470 ) ;
#6697=VERTEX_POINT ( 'NONE', #175 ) ;
#6702=EDGE_CURVE ( 'NONE', #16262, #6658, #21934, .T. ) ;
#6738=CARTESIAN_POINT ( 'NONE',  ( -18.35824191589999899, -1.500000000000000000, -142.9407682190000060 ) ) ;
#6741=VERTEX_POINT ( 'NONE', #20632 ) ;
#6745=ORIENTED_EDGE ( 'NONE', *, *, #17409, .F. ) ;
#6758=CARTESIAN_POINT ( 'NONE',  ( 10.68320006080000084, -20.50000000000000000, -150.0552959529999839 ) ) ;
#6761=VECTOR ( 'NONE', #42, 1000.000000000000000 ) ;
#6768=EDGE_CURVE ( 'NONE', #17007, #21283, #887, .T. ) ;
#6777=CARTESIAN_POINT ( 'NONE',  ( -18.35824191589999899, -34.50000000000000000, -148.1907682189999775 ) ) ;
#6781=DIRECTION ( 'NONE',  ( -0.7071067811865475727, 0.7071067811865475727, 0.000000000000000000 ) ) ;
#6793=CARTESIAN_POINT ( 'NONE',  ( -18.07392865170000107, -34.50000000000000000, -147.3157682190000060 ) ) ;
#6796=ORIENTED_EDGE ( 'NONE', *, *, #1963, .F. ) ;
#6824=CIRCLE ( 'NONE', #11749, 2.499999999999998668 ) ;
#6829=DIRECTION ( 'NONE',  ( 0.000000000000000000, -4.148443855749999753E-27, -1.000000000000000000 ) ) ;
#6848=EDGE_LOOP ( 'NONE', ( #12403, #8508, #18544, #10206 ) ) ;
#6850=EDGE_CURVE ( 'NONE', #16441, #12024, #13362, .T. ) ;
#6871=CARTESIAN_POINT ( 'NONE',  ( -17.08727435560000174, -34.50000000000000000, -147.1525923079999814 ) ) ;
#6882=DIRECTION ( 'NONE',  ( 1.211690350419999855E-27, 2.765629237170000203E-27, -1.000000000000000000 ) ) ;
#6888=AXIS2_PLACEMENT_3D ( 'NONE', #6315, #15366, #2766 ) ;
#6890=ORIENTED_EDGE ( 'NONE', *, *, #16204, .F. ) ;
#6891=CARTESIAN_POINT ( 'NONE',  ( 0.1832000607640000001, -6.500000000000000000, -149.3052959529999839 ) ) ;
#6892=FACE_BOUND ( 'NONE', #10820, .T. ) ;
#6897=LINE ( 'NONE', #10101, #4772 ) ;
#6900=DIRECTION ( 'NONE',  ( 0.000000000000000000, -4.148443855749999753E-27, -1.000000000000000000 ) ) ;
#6901=DIRECTION ( 'NONE',  ( 1.000000000000000000, 0.000000000000000000, 0.000000000000000000 ) ) ;
#6909=DIRECTION ( 'NONE',  ( 1.000000000000000000, 0.000000000000000000, 2.506439500389999993E-12 ) ) ;
#6913=FACE_OUTER_BOUND ( 'NONE', #20084, .T. ) ;
#6920=AXIS2_PLACEMENT_3D ( 'NONE', #11163, #21904, #11051 ) ;
#6925=CIRCLE ( 'NONE', #21000, 0.7500000000000006661 ) ;
#6944=EDGE_LOOP ( 'NONE', ( #5453, #20053, #10536, #3422 ) ) ;
#6977=VERTEX_POINT ( 'NONE', #8817 ) ;
#6982=DIRECTION ( 'NONE',  ( 2.506794771760000178E-12, 5.921189464669999937E-17, -1.000000000000000000 ) ) ;
#6983=DIRECTION ( 'NONE',  ( 1.000000000000000000, 0.000000000000000000, 2.516505522483685870E-12 ) ) ;
#7007=AXIS2_PLACEMENT_3D ( 'NONE', #21208, #22741, #5018 ) ;
#7024=LINE ( 'NONE', #14536, #9824 ) ;
#7028=CARTESIAN_POINT ( 'NONE',  ( -21.35824191589999899, -32.00000000000000000, -146.2257682199999920 ) ) ;
#7029=DIRECTION ( 'NONE',  ( 1.000000000000000000, 0.000000000000000000, 2.516505522483685870E-12 ) ) ;
#7036=VERTEX_POINT ( 'NONE', #5607 ) ;
#7044=EDGE_CURVE ( 'NONE', #5708, #10881, #2296, .T. ) ;
#7052=ADVANCED_FACE ( 'NONE', ( #16552 ), #7621, .T. ) ;
#7055=CARTESIAN_POINT ( 'NONE',  ( -21.35824191591069265, -4.000000000000000000, -141.9623572383524959 ) ) ;
#7063=EDGE_LOOP ( 'NONE', ( #2861, #6023, #3078, #12633 ) ) ;
#7099=AXIS2_PLACEMENT_3D ( 'NONE', #9196, #176, #1737 ) ;
#7101=FACE_OUTER_BOUND ( 'NONE', #21443, .T. ) ;
#7126=VECTOR ( 'NONE', #4185, 1000.000000000000000 ) ;
#7131=CARTESIAN_POINT ( 'NONE',  ( 10.93320006080000084, -15.50000000000000000, -150.0552959529999839 ) ) ;
#7140=VERTEX_POINT ( 'NONE', #2864 ) ;
#7149=CARTESIAN_POINT ( 'NONE',  ( -18.35824191589999899, -1.500000000000000000, -148.1907682189999775 ) ) ;
#7161=ORIENTED_EDGE ( 'NONE', *, *, #22668, .T. ) ;
#7178=EDGE_CURVE ( 'NONE', #19530, #11089, #12058, .T. ) ;
#7180=PLANE ( 'NONE',  #4581 ) ;
#7197=VERTEX_POINT ( 'NONE', #8195 ) ;
#7201=EDGE_CURVE ( 'NONE', #20840, #10047, #7847, .T. ) ;
#7202=ORIENTED_EDGE ( 'NONE', *, *, #12190, .F. ) ;
#7206=LINE ( 'NONE', #19827, #2072 ) ;
#7219=AXIS2_PLACEMENT_3D ( 'NONE', #19453, #4575, #8487 ) ;
#7230=VERTEX_POINT ( 'NONE', #20483 ) ;
#7232=EDGE_CURVE ( 'NONE', #963, #4709, #11890, .T. ) ;
#7248=CARTESIAN_POINT ( 'NONE',  ( -14.47770030809999930, -18.00000000000000000, -150.0552959529999839 ) ) ;
#7253=CARTESIAN_POINT ( 'NONE',  ( -20.62738678477109744, -4.195399377771871663, -146.3157682190057187 ) ) ;
#7269=VECTOR ( 'NONE', #9449, 1000.000000000000000 ) ;
#7271=CLOSED_SHELL ( 'NONE', ( #394, #22310, #6502, #13035, #11291, #2332 ) ) ;
#7293=ADVANCED_FACE ( 'NONE', ( #20104, #1792, #21897 ), #7370, .F. ) ;
#7294=FACE_OUTER_BOUND ( 'NONE', #19218, .T. ) ;
#7299=ORIENTED_EDGE ( 'NONE', *, *, #8346, .T. ) ;
#7316=ADVANCED_FACE ( 'NONE', ( #18430 ), #5810, .F. ) ;
#7330=ORIENTED_EDGE ( 'NONE', *, *, #22193, .T. ) ;
#7364=LINE ( 'NONE', #465, #14797 ) ;
#7370=PLANE ( 'NONE',  #15868 ) ;
#7381=LINE ( 'NONE', #16195, #13701 ) ;
#7389=VERTEX_POINT ( 'NONE', #2600 ) ;
#7390=PRODUCT_DEFINITION_SHAPE ( 'NONE', 'NONE',  #10930 ) ;
#7401=DIRECTION ( 'NONE',  ( -3.994014902950000436E-29, 1.000000000000000000, -4.148443855749999753E-27 ) ) ;
#7419=COLOUR_RGB ( '', 0.09019608, 0.27058824, 0.51372549) ;
#7420=DIRECTION ( 'NONE',  ( 2.507771768019999718E-12, 1.592654864209999947E-17, -1.000000000000000000 ) ) ;
#7425=ORIENTED_EDGE ( 'NONE', *, *, #18621, .F. ) ;
#7453=ORIENTED_EDGE ( 'NONE', *, *, #5055, .T. ) ;
#7472=CARTESIAN_POINT ( 'NONE',  ( -20.75825067126470813, -4.460833112886678720, -146.3157682190060029 ) ) ;
#7476=CIRCLE ( 'NONE', #1420, 0.7500000000000006661 ) ;
#7479=CYLINDRICAL_SURFACE ( 'NONE', #12762, 0.7500000000000006661 ) ;
#7491=DIRECTION ( 'NONE',  ( 1.000000000000000000, 0.000000000000000000, 0.000000000000000000 ) ) ;
#7497=EDGE_CURVE ( 'NONE', #13760, #18415, #9783, .T. ) ;
#7549=DIRECTION ( 'NONE',  ( -0.1736481776649230202, 0.000000000000000000, 0.9848077530125619594 ) ) ;
#7571=ORIENTED_EDGE ( 'NONE', *, *, #8062, .F. ) ;
#7574=CARTESIAN_POINT ( 'NONE',  ( -25.85824191589999899, -1.500000000000000000, -145.5657682190000060 ) ) ;
#7580=DIRECTION ( 'NONE',  ( -1.211690350418039921E-27, -2.765629237168040089E-27, 1.000000000000000000 ) ) ;
#7585=DIRECTION ( 'NONE',  ( 1.000000000000000000, 0.000000000000000000, 2.516505522483685870E-12 ) ) ;
#7588=CARTESIAN_POINT ( 'NONE',  ( 14.79224200840030257, -34.50000000000000000, -149.4708568728852356 ) ) ;
#7594=DIRECTION ( 'NONE',  ( -3.994014902950000436E-29, 1.000000000000000000, -4.148443855750100198E-27 ) ) ;
#7610=DIRECTION ( 'NONE',  ( -1.000000000000000000, 0.000000000000000000, -2.516505522483685870E-12 ) ) ;
#7621=PLANE ( 'NONE',  #17384 ) ;
#7626=DIRECTION ( 'NONE',  ( -1.211690350418039921E-27, -2.765629237168040089E-27, 1.000000000000000000 ) ) ;
#7633=FACE_OUTER_BOUND ( 'NONE', #14373, .T. ) ;
#7645=ORIENTED_EDGE ( 'NONE', *, *, #20346, .F. ) ;
#7648=ADVANCED_FACE ( 'NONE', ( #20285 ), #3979, .F. ) ;
#7659=ORIENTED_EDGE ( 'NONE', *, *, #2129, .F. ) ;
#7692=DIRECTION ( 'NONE',  ( -2.808280234682504769E-18, 1.000000000000000000, 1.592654863660134930E-17 ) ) ;
#7695=CARTESIAN_POINT ( 'NONE',  ( 10.93320006080000084, 3.500000000000000000, -148.5552959529999839 ) ) ;
#7702=CARTESIAN_POINT ( 'NONE',  ( -16.35051508389999597, -34.50000000000000000, -147.0118839079999873 ) ) ;
#7704=VERTEX_POINT ( 'NONE', #1603 ) ;
#7729=CARTESIAN_POINT ( 'NONE',  ( 11.55556760165677233, -19.99386613923380906, -148.5552959529999839 ) ) ;
#7731=ORIENTED_EDGE ( 'NONE', *, *, #3277, .T. ) ;
#7750=CARTESIAN_POINT ( 'NONE',  ( -18.35824191589999899, -34.50000000000000000, -144.8157682189915931 ) ) ;
#7776=ADVANCED_FACE ( 'NONE', ( #16450 ), #22157, .F. ) ;
#7785=EDGE_CURVE ( 'NONE', #3040, #22250, #5503, .T. ) ;
#7787=LINE ( 'NONE', #20308, #16984 ) ;
#7793=CIRCLE ( 'NONE', #6666, 0.7500000000000006661 ) ;
#7794=ORIENTED_EDGE ( 'NONE', *, *, #17409, .T. ) ;
#7816=PLANE ( 'NONE',  #2263 ) ;
#7817=ORIENTED_EDGE ( 'NONE', *, *, #20743, .T. ) ;
#7844=CARTESIAN_POINT ( 'NONE',  ( -20.60824191589623666, -32.00000000000000000, -146.3157682190056335 ) ) ;
#7847=LINE ( 'NONE', #15467, #1432 ) ;
#7869=CARTESIAN_POINT ( 'NONE',  ( -7.816799939239999162, 0.9999999999989999111, -149.3052959529999839 ) ) ;
#7870=VERTEX_POINT ( 'NONE', #9398 ) ;
#7878=EDGE_CURVE ( 'NONE', #21963, #3124, #5614, .T. ) ;
#7881=CYLINDRICAL_SURFACE ( 'NONE', #9239, 0.7499999999999997780 ) ;
#7892=ADVANCED_FACE ( 'NONE', ( #12989 ), #20263, .F. ) ;
#7896=DIRECTION ( 'NONE',  ( -1.000000000000000000, 0.000000000000000000, -2.508689552389999873E-12 ) ) ;
#7908=ORIENTED_EDGE ( 'NONE', *, *, #14188, .T. ) ;
#7914=ORIENTED_EDGE ( 'NONE', *, *, #19917, .F. ) ;
#7919=FACE_OUTER_BOUND ( 'NONE', #15145, .T. ) ;
#7941=PLANE ( 'NONE',  #19469 ) ;
#7948=PLANE ( 'NONE',  #20203 ) ;
#7957=DIRECTION ( 'NONE',  ( -2.507771768020000122E-12, -0.000000000000000000, 1.000000000000000000 ) ) ;
#7970=CARTESIAN_POINT ( 'NONE',  ( -20.60824191589811605, -4.000000000000000000, -146.3157682190056335 ) ) ;
#7978=FACE_OUTER_BOUND ( 'NONE', #15437, .T. ) ;
#7981=VECTOR ( 'NONE', #5941, 1000.000000000000000 ) ;
#7982=VECTOR ( 'NONE', #19711, 1000.000000000000000 ) ;
#8007=EDGE_LOOP ( 'NONE', ( #654, #17705, #9921, #4372 ) ) ;
#8008=DIRECTION ( 'NONE',  ( -1.000000000000000000, -2.808280234649999694E-18, -2.507771768019999718E-12 ) ) ;
#8016=CARTESIAN_POINT ( 'NONE',  ( 0.3832000607639999834, -24.50000000000000000, -148.5552959529999839 ) ) ;
#8031=ADVANCED_FACE ( 'NONE', ( #19764 ), #14398, .F. ) ;
#8039=( NAMED_UNIT ( * ) PLANE_ANGLE_UNIT ( ) SI_UNIT ( $, .RADIAN. ) );
#8043=EDGE_LOOP ( 'NONE', ( #19085, #19849, #20706, #4833 ) ) ;
#8052=ORIENTED_EDGE ( 'NONE', *, *, #16575, .T. ) ;
#8062=EDGE_CURVE ( 'NONE', #3729, #2396, #1573, .T. ) ;
#8067=VECTOR ( 'NONE', #17327, 1000.000000000000000 ) ;
#8077=ADVANCED_FACE ( 'NONE', ( #21674 ), #17855, .T. ) ;
#8088=CARTESIAN_POINT ( 'NONE',  ( -20.68907173818941203, -3.608510005926304665, -146.3157682189983007 ) ) ;
#8095=FACE_OUTER_BOUND ( 'NONE', #16995, .T. ) ;
#8097=CARTESIAN_POINT ( 'NONE',  ( -21.35824191589999899, -4.000000000000000000, -146.2257682199999920 ) ) ;
#8099=CARTESIAN_POINT ( 'NONE',  ( 11.68320006079999906, -20.50000000000000000, -149.3052959529999839 ) ) ;
#8106=DIRECTION ( 'NONE',  ( -3.994014902950000436E-29, 1.000000000000000000, -4.148443855749999753E-27 ) ) ;
#8123=LINE ( 'NONE', #4451, #19139 ) ;
#8147=VERTEX_POINT ( 'NONE', #3332 ) ;
#8159=ORIENTED_CLOSED_SHELL ( 'NONE', *, #7271, .F. );
#8164=DIRECTION ( 'NONE',  ( 1.211690350419999855E-27, 2.765629237170000203E-27, -1.000000000000000000 ) ) ;
#8166=CARTESIAN_POINT ( 'NONE',  ( 29.68320006080000084, -7.750000000000000000, -148.5552959529999839 ) ) ;
#8187=DIRECTION ( 'NONE',  ( 1.000000000000000000, 0.000000000000000000, 2.507771768019999718E-12 ) ) ;
#8188=DIRECTION ( 'NONE',  ( 1.000000000000000000, 0.000000000000000000, 0.000000000000000000 ) ) ;
#8195=CARTESIAN_POINT ( 'NONE',  ( -20.60824191589186327, -32.00000000000000000, -149.4708568729739966 ) ) ;
#8207=EDGE_CURVE ( 'NONE', #22041, #8776, #18545, .T. ) ;
#8224=CARTESIAN_POINT ( 'NONE',  ( -22.10824191590187837, -4.000000000000000000, -144.8157682189905984 ) ) ;
#8237=SURFACE_STYLE_USAGE ( .BOTH. , #12780 ) ;
#8252=APPLICATION_CONTEXT ( 'automotive_design' ) ;
#8258=UNCERTAINTY_MEASURE_WITH_UNIT (LENGTH_MEASURE( 1.000000000000000082E-05 ), #2820, 'distance_accuracy_value', 'NONE');
#8273=CARTESIAN_POINT ( 'NONE',  ( 0.1832000610750000313, -6.500000000000000000, -150.0552959529999839 ) ) ;
#8284=DIRECTION ( 'NONE',  ( -2.507771768019999718E-12, -1.592654864209999947E-17, 1.000000000000000000 ) ) ;
#8285=FACE_OUTER_BOUND ( 'NONE', #8766, .T. ) ;
#8290=VERTEX_POINT ( 'NONE', #9144 ) ;
#8314=DIRECTION ( 'NONE',  ( 0.000000000000000000, -1.000000000000000000, -1.592654864069999939E-17 ) ) ;
#8328=ORIENTED_EDGE ( 'NONE', *, *, #768, .T. ) ;
#8335=AXIS2_PLACEMENT_3D ( 'NONE', #14246, #5082, #6983 ) ;
#8342=DIRECTION ( 'NONE',  ( 1.000000000000000000, 0.000000000000000000, 0.000000000000000000 ) ) ;
#8346=EDGE_CURVE ( 'NONE', #17007, #22008, #6824, .T. ) ;
#8360=CIRCLE ( 'NONE', #20916, 2.500000000000000444 ) ;
#8364=EDGE_CURVE ( 'NONE', #8849, #8147, #6169, .T. ) ;
#8381=AXIS2_PLACEMENT_3D ( 'NONE', #3377, #16232, #12295 ) ;
#8398=ORIENTED_EDGE ( 'NONE', *, *, #1957, .T. ) ;
#8411=VECTOR ( 'NONE', #15183, 1000.000000000000000 ) ;
#8437=ADVANCED_FACE ( 'NONE', ( #15094, #20933, #11867 ), #13306, .T. ) ;
#8439=CARTESIAN_POINT ( 'NONE',  ( 24.68320006080000084, -16.50000000000000000, -148.5552959529999839 ) ) ;
#8440=FACE_OUTER_BOUND ( 'NONE', #702, .T. ) ;
#8472=EDGE_LOOP ( 'NONE', ( #23246, #4492, #6571, #22154 ) ) ;
#8484=DIRECTION ( 'NONE',  ( 1.000000000000000000, 0.000000000000000000, 2.504935852220000146E-12 ) ) ;
#8487=DIRECTION ( 'NONE',  ( -1.000000000000000000, -3.994014902950000436E-29, 0.000000000000000000 ) ) ;
#8489=ORIENTED_EDGE ( 'NONE', *, *, #4333, .F. ) ;
#8495=ADVANCED_FACE ( 'NONE', ( #17703 ), #12101, .F. ) ;
#8508=ORIENTED_EDGE ( 'NONE', *, *, #17066, .F. ) ;
#8515=DIRECTION ( 'NONE',  ( 2.507554887169999917E-12, 0.000000000000000000, -1.000000000000000000 ) ) ;
#8531=ADVANCED_FACE ( 'NONE', ( #1192 ), #8638, .T. ) ;
#8536=CARTESIAN_POINT ( 'NONE',  ( -21.35824191589811605, -3.250000000000000000, -146.3157682190075093 ) ) ;
#8542=VECTOR ( 'NONE', #126, 1000.000000000000000 ) ;
#8562=DIRECTION ( 'NONE',  ( -2.507771768019999718E-12, -1.592654864069999939E-17, 1.000000000000000000 ) ) ;
#8567=ORIENTED_EDGE ( 'NONE', *, *, #6850, .T. ) ;
#8588=AXIS2_PLACEMENT_3D ( 'NONE', #13205, #2294, #2517 ) ;
#8638=PLANE ( 'NONE',  #9082 ) ;
#8640=VERTEX_POINT ( 'NONE', #21127 ) ;
#8670=EDGE_LOOP ( 'NONE', ( #1887, #13574, #9737, #16965 ) ) ;
#8682=VECTOR ( 'NONE', #1911, 1000.000000000000000 ) ;
#8690=DIRECTION ( 'NONE',  ( -2.508215857230000030E-12, 0.000000000000000000, 1.000000000000000000 ) ) ;
#8694=ORIENTED_EDGE ( 'NONE', *, *, #5736, .T. ) ;
#8714=ORIENTED_EDGE ( 'NONE', *, *, #22483, .F. ) ;
#8727=AXIS2_PLACEMENT_3D ( 'NONE', #20882, #8008, #15292 ) ;
#8750=EDGE_CURVE ( 'NONE', #10047, #16262, #1493, .T. ) ;
#8751=LINE ( 'NONE', #6738, #365 ) ;
#8766=EDGE_LOOP ( 'NONE', ( #11872, #13724, #11382, #23272 ) ) ;
#8771=DIRECTION ( 'NONE',  ( 1.000000000000000000, 0.000000000000000000, 2.507771768020000122E-12 ) ) ;
#8776=VERTEX_POINT ( 'NONE', #20389 ) ;
#8778=AXIS2_PLACEMENT_3D ( 'NONE', #5390, #12637, #19908 ) ;
#8780=VERTEX_POINT ( 'NONE', #20166 ) ;
#8789=ADVANCED_FACE ( 'NONE', ( #18477 ), #22175, .F. ) ;
#8796=AXIS2_PLACEMENT_3D ( 'NONE', #11903, #4419, #9878 ) ;
#8809=EDGE_CURVE ( 'NONE', #19622, #1286, #6469, .T. ) ;
#8817=CARTESIAN_POINT ( 'NONE',  ( -25.85824191589999899, -34.50000000000000000, -144.8157682190000060 ) ) ;
#8828=ORIENTED_EDGE ( 'NONE', *, *, #2649, .F. ) ;
#8837=EDGE_LOOP ( 'NONE', ( #15261, #18588, #9838, #15070 ) ) ;
#8849=VERTEX_POINT ( 'NONE', #22061 ) ;
#8860=ORIENTED_EDGE ( 'NONE', *, *, #6702, .F. ) ;
#8878=ORIENTED_EDGE ( 'NONE', *, *, #9936, .T. ) ;
#8897=ORIENTED_EDGE ( 'NONE', *, *, #22917, .T. ) ;
#8906=CARTESIAN_POINT ( 'NONE',  ( -16.93971969060000049, -18.00000000000000000, -147.9894163970000136 ) ) ;
#8907=DIRECTION ( 'NONE',  ( 1.110223024629999900E-16, -1.000000000000000000, 4.148443855749999753E-27 ) ) ;
#8937=DIRECTION ( 'NONE',  ( 0.000000000000000000, -4.148443855749999753E-27, -1.000000000000000000 ) ) ;
#8938=EDGE_CURVE ( 'NONE', #3553, #16262, #12578, .T. ) ;
#8944=DIRECTION ( 'NONE',  ( 1.000000000000000000, 0.000000000000000000, 2.516505522483685870E-12 ) ) ;
#8974=CARTESIAN_POINT ( 'NONE',  ( -22.10824191589999899, -4.000000000000000000, -150.0657682190000060 ) ) ;
#9004=CARTESIAN_POINT ( 'NONE',  ( 10.68320006080000084, -20.50000000000000000, -150.0552959529999839 ) ) ;
#9006=FACE_OUTER_BOUND ( 'NONE', #15975, .T. ) ;
#9016=VERTEX_POINT ( 'NONE', #22448 ) ;
#9018=CARTESIAN_POINT ( 'NONE',  ( -21.35824191589999899, -4.000000000000000000, -146.2257682199999920 ) ) ;
#9022=CARTESIAN_POINT ( 'NONE',  ( -22.10824191589999899, -32.00000000000000000, -146.3157682190000060 ) ) ;
#9053=PLANE ( 'NONE',  #847 ) ;
#9077=VERTEX_POINT ( 'NONE', #5790 ) ;
#9082=AXIS2_PLACEMENT_3D ( 'NONE', #6871, #15913, #10318 ) ;
#9084=ORIENTED_EDGE ( 'NONE', *, *, #5963, .F. ) ;
#9087=EDGE_LOOP ( 'NONE', ( #9683, #7202, #6796, #11804 ) ) ;
#9090=ORIENTED_EDGE ( 'NONE', *, *, #22483, .T. ) ;
#9097=ORIENTED_EDGE ( 'NONE', *, *, #8207, .T. ) ;
#9104=DIRECTION ( 'NONE',  ( 0.000000000000000000, 0.000000000000000000, 1.000000000000000000 ) ) ;
#9136=PLANE ( 'NONE',  #5204 ) ;
#9144=CARTESIAN_POINT ( 'NONE',  ( 10.68320006080000084, -19.50000000000000000, -148.5552959529999839 ) ) ;
#9163=ORIENTED_EDGE ( 'NONE', *, *, #15905, .F. ) ;
#9166=CARTESIAN_POINT ( 'NONE',  ( 9.683200060759999062, -20.50000000000000000, -149.3052959529999839 ) ) ;
#9167=DIRECTION ( 'NONE',  ( 1.000000000000000000, 0.000000000000000000, 2.516505522483685870E-12 ) ) ;
#9186=VECTOR ( 'NONE', #15371, 1000.000000000000227 ) ;
#9193=DIRECTION ( 'NONE',  ( 1.000000000000000000, 0.000000000000000000, 0.000000000000000000 ) ) ;
#9196=CARTESIAN_POINT ( 'NONE',  ( -21.35824191589999899, -32.00000000000000000, -150.0657682190000060 ) ) ;
#9231=EDGE_CURVE ( 'NONE', #7230, #15557, #19700, .T. ) ;
#9239=AXIS2_PLACEMENT_3D ( 'NONE', #2552, #11213, #20288 ) ;
#9245=DIRECTION ( 'NONE',  ( -0.9836666101882604041, 0.000000000000000000, -0.1800000000020474666 ) ) ;
#9271=LINE ( 'NONE', #10580, #13087 ) ;
#9273=VECTOR ( 'NONE', #9879, 1000.000000000000000 ) ;
#9289=CARTESIAN_POINT ( 'NONE',  ( 10.17706620004303986, -19.62763245910807797, -148.5552959529999839 ) ) ;
#9305=CARTESIAN_POINT ( 'NONE',  ( -15.31679993919999916, -34.50000000000000000, -150.0552959529999839 ) ) ;
#9311=( NAMED_UNIT ( * ) SI_UNIT ( $, .STERADIAN. ) SOLID_ANGLE_UNIT ( ) );
#9325=CARTESIAN_POINT ( 'NONE',  ( 18.18320006080000084, 0.4999999999990000776, -150.0552959529999839 ) ) ;
#9330=VECTOR ( 'NONE', #8690, 1000.000000000000000 ) ;
#9350=DIRECTION ( 'NONE',  ( 0.7071067811865475727, 0.7071067811865475727, 0.000000000000000000 ) ) ;
#9367=CARTESIAN_POINT ( 'NONE',  ( -20.60824191589999899, -4.000000000000000000, -146.2257682199999920 ) ) ;
#9368=DIRECTION ( 'NONE',  ( -2.508215857230000030E-12, 0.000000000000000000, 1.000000000000000000 ) ) ;
#9382=EDGE_CURVE ( 'NONE', #10546, #22041, #2251, .T. ) ;
#9398=CARTESIAN_POINT ( 'NONE',  ( -25.85824191589999899, -1.500000000000000000, -144.8157682190000060 ) ) ;
#9427=ORIENTED_EDGE ( 'NONE', *, *, #8364, .T. ) ;
#9429=CARTESIAN_POINT ( 'NONE',  ( -18.35824191589999899, -34.50000000000000000, -144.8157682190000060 ) ) ;
#9430=DIRECTION ( 'NONE',  ( 1.000000000000000000, 0.000000000000000000, 0.000000000000000000 ) ) ;
#9443=CARTESIAN_POINT ( 'NONE',  ( -18.07392865170000107, -1.500000000000000000, -145.5657682190000060 ) ) ;
#9449=DIRECTION ( 'NONE',  ( -1.000000000000000000, 0.000000000000000000, 0.000000000000000000 ) ) ;
#9508=ORIENTED_EDGE ( 'NONE', *, *, #11064, .F. ) ;
#9519=ORIENTED_EDGE ( 'NONE', *, *, #8809, .T. ) ;
#9527=VECTOR ( 'NONE', #12677, 1000.000000000000000 ) ;
#9547=DIRECTION ( 'NONE',  ( 0.000000000000000000, -1.000000000000000000, 0.000000000000000000 ) ) ;
#9555=ORIENTED_EDGE ( 'NONE', *, *, #3025, .T. ) ;
#9561=DIRECTION ( 'NONE',  ( 0.000000000000000000, 0.000000000000000000, 1.000000000000000000 ) ) ;
#9574=LINE ( 'NONE', #10264, #8411 ) ;
#9575=ORIENTED_EDGE ( 'NONE', *, *, #22935, .T. ) ;
#9590=AXIS2_PLACEMENT_3D ( 'NONE', #6793, #3591, #5599 ) ;
#9596=DIRECTION ( 'NONE',  ( 2.507554887169999917E-12, 0.000000000000000000, -1.000000000000000000 ) ) ;
#9598=EDGE_LOOP ( 'NONE', ( #12233, #1008, #5665, #21862 ) ) ;
#9605=EDGE_CURVE ( 'NONE', #11959, #8849, #7024, .T. ) ;
#9608=CYLINDRICAL_SURFACE ( 'NONE', #6920, 0.7500000000000006661 ) ;
#9619=CARTESIAN_POINT ( 'NONE',  ( -21.55459145674873866, -4.749999999999015010, -146.3157682190004891 ) ) ;
#9621=CARTESIAN_POINT ( 'NONE',  ( 10.94417203217891021, -19.52598336879741936, -148.5552959530000123 ) ) ;
#9623=ORIENTED_EDGE ( 'NONE', *, *, #15028, .T. ) ;
#9626=CYLINDRICAL_SURFACE ( 'NONE', #8588, 0.7500000000000006661 ) ;
#9641=CARTESIAN_POINT ( 'NONE',  ( -7.816799939239999162, -0.2500000000010000334, -148.5552959529999839 ) ) ;
#9650=EDGE_CURVE ( 'NONE', #15634, #10783, #12487, .T. ) ;
#9660=CARTESIAN_POINT ( 'NONE',  ( 12.68320006080000084, -24.50000000000000000, -149.3052959529999839 ) ) ;
#9662=EDGE_LOOP ( 'NONE', ( #2011, #16586, #15484, #16108 ) ) ;
#9683=ORIENTED_EDGE ( 'NONE', *, *, #11345, .T. ) ;
#9704=DIRECTION ( 'NONE',  ( -2.507771768019999718E-12, -1.592654864069999939E-17, 1.000000000000000000 ) ) ;
#9717=CARTESIAN_POINT ( 'NONE',  ( -25.35824191590000254, -18.00000000000000000, -144.8157682190000060 ) ) ;
#9732=CARTESIAN_POINT ( 'NONE',  ( 10.68320006080000084, -19.50000000000000000, -148.5552959529999839 ) ) ;
#9737=ORIENTED_EDGE ( 'NONE', *, *, #2558, .F. ) ;
#9750=VECTOR ( 'NONE', #5061, 1000.000000000000000 ) ;
#9751=CARTESIAN_POINT ( 'NONE',  ( -14.47770030809999930, -34.50000000000000000, -147.5552959529999839 ) ) ;
#9761=CARTESIAN_POINT ( 'NONE',  ( 0.1832000607640000001, -3.000000000000000000, -148.5552959529999839 ) ) ;
#9781=CARTESIAN_POINT ( 'NONE',  ( -11.14725012360000100, -1.500000000000000000, -148.5552959529999839 ) ) ;
#9783=CIRCLE ( 'NONE', #15123, 0.7500000000000006661 ) ;
#9786=CARTESIAN_POINT ( 'NONE',  ( -14.47770030809999930, -1.500000000000000000, -147.5552959529999839 ) ) ;
#9796=EDGE_CURVE ( 'NONE', #21283, #18104, #10208, .T. ) ;
#9798=AXIS2_PLACEMENT_3D ( 'NONE', #11033, #5682, #11145 ) ;
#9805=ORIENTED_EDGE ( 'NONE', *, *, #12624, .F. ) ;
#9811=ORIENTED_EDGE ( 'NONE', *, *, #12973, .T. ) ;
#9817=( NAMED_UNIT ( * ) SI_UNIT ( $, .STERADIAN. ) SOLID_ANGLE_UNIT ( ) );
#9824=VECTOR ( 'NONE', #12490, 1000.000000000000000 ) ;
#9833=DIRECTION ( 'NONE',  ( -2.509104035652851358E-12, 0.000000000000000000, 1.000000000000000000 ) ) ;
#9838=ORIENTED_EDGE ( 'NONE', *, *, #3884, .T. ) ;
#9846=FACE_OUTER_BOUND ( 'NONE', #13128, .T. ) ;
#9850=CIRCLE ( 'NONE', #23170, 0.7500000000000006661 ) ;
#9856=DIRECTION ( 'NONE',  ( -1.734723475976805517E-14, -1.000000000000000000, 0.000000000000000000 ) ) ;
#9872=EDGE_CURVE ( 'NONE', #6188, #5644, #13251, .T. ) ;
#9878=DIRECTION ( 'NONE',  ( 1.000000000000000000, 0.000000000000000000, 0.000000000000000000 ) ) ;
#9879=DIRECTION ( 'NONE',  ( 0.000000000000000000, 0.000000000000000000, 1.000000000000000000 ) ) ;
#9890=DIRECTION ( 'NONE',  ( 2.507771768019999718E-12, 1.592654864069999939E-17, -1.000000000000000000 ) ) ;
#9910=CIRCLE ( 'NONE', #13339, 3.499999999999999556 ) ;
#9921=ORIENTED_EDGE ( 'NONE', *, *, #19681, .T. ) ;
#9927=ORIENTED_EDGE ( 'NONE', *, *, #3251, .F. ) ;
#9931=VERTEX_POINT ( 'NONE', #8536 ) ;
#9933=EDGE_LOOP ( 'NONE', ( #18784, #20954, #17941, #21567 ) ) ;
#9936=EDGE_CURVE ( 'NONE', #19743, #10194, #19762, .T. ) ;
#9954=PLANE ( 'NONE',  #1583 ) ;
#9967=ORIENTED_EDGE ( 'NONE', *, *, #10137, .F. ) ;
#9968=DIRECTION ( 'NONE',  ( 2.507771768019999718E-12, 1.592654864209999947E-17, -1.000000000000000000 ) ) ;
#9973=FACE_BOUND ( 'NONE', #14182, .T. ) ;
#9980=CARTESIAN_POINT ( 'NONE',  ( 0.1832000607640000001, 0.4999999999990000776, -150.0552959529999839 ) ) ;
#9994=CARTESIAN_POINT ( 'NONE',  ( -21.35824191589999899, -4.000000000000000000, -144.8157682190000060 ) ) ;
#10000=CARTESIAN_POINT ( 'NONE',  ( -21.35824191589999899, -32.75000000000000000, -146.3157682190075093 ) ) ;
#10021=DIRECTION ( 'NONE',  ( -1.000000000000000000, 0.000000000000000000, -2.516505522483685870E-12 ) ) ;
#10022=CARTESIAN_POINT ( 'NONE',  ( 10.68320006080000084, -21.50000000000000000, -148.5552959529999839 ) ) ;
#10037=DIRECTION ( 'NONE',  ( -2.507771768023035002E-12, -1.592654560756634986E-17, 1.000000000000000000 ) ) ;
#10046=ADVANCED_BREP_SHAPE_REPRESENTATION ( '', ( #4113, #5025 ), #5047 ) ;
#10047=VERTEX_POINT ( 'NONE', #18068 ) ;
#10050=CYLINDRICAL_SURFACE ( 'NONE', #22525, 2.500000000000000000 ) ;
#10057=CYLINDRICAL_SURFACE ( 'NONE', #3019, 2.499999999999998668 ) ;
#10064=ORIENTED_EDGE ( 'NONE', *, *, #3720, .F. ) ;
#10090=EDGE_LOOP ( 'NONE', ( #7731, #7330 ) ) ;
#10101=CARTESIAN_POINT ( 'NONE',  ( -22.10824191589999899, -34.50000000000000000, -144.8157682190000060 ) ) ;
#10102=EDGE_CURVE ( 'NONE', #7870, #3729, #12935, .T. ) ;
#10108=CARTESIAN_POINT ( 'NONE',  ( 0.1832000607640000001, 0.4999999999990000776, -148.5552959529999839 ) ) ;
#10130=CARTESIAN_POINT ( 'NONE',  ( -25.35824191590000254, -34.50000000000000000, -144.8157682190000060 ) ) ;
#10137=EDGE_CURVE ( 'NONE', #2396, #17085, #16971, .T. ) ;
#10146=ORIENTED_EDGE ( 'NONE', *, *, #4143, .T. ) ;
#10153=CARTESIAN_POINT ( 'NONE',  ( 12.68320006090000085, -24.50000000000000000, -150.0552959529999839 ) ) ;
#10158=DIRECTION ( 'NONE',  ( -1.000000000000000000, 0.000000000000000000, 0.000000000000000000 ) ) ;
#10194=VERTEX_POINT ( 'NONE', #21263 ) ;
#10203=DIRECTION ( 'NONE',  ( 1.000000000000000000, 0.000000000000000000, 2.516505522483685870E-12 ) ) ;
#10206=ORIENTED_EDGE ( 'NONE', *, *, #15367, .T. ) ;
#10208=CIRCLE ( 'NONE', #11336, 2.499999999999998668 ) ;
#10222=VERTEX_POINT ( 'NONE', #11961 ) ;
#10232=ORIENTED_EDGE ( 'NONE', *, *, #3703, .F. ) ;
#10245=AXIS2_PLACEMENT_3D ( 'NONE', #3258, #5273, #21715 ) ;
#10259=CARTESIAN_POINT ( 'NONE',  ( -12.87073128380000142, -34.50000000000000000, -149.4704070610000031 ) ) ;
#10264=CARTESIAN_POINT ( 'NONE',  ( 10.68320006080000084, -21.50000000000000000, -149.3052959529999839 ) ) ;
#10267=CIRCLE ( 'NONE', #413, 3.499999999999999556 ) ;
#10275=FACE_OUTER_BOUND ( 'NONE', #5670, .T. ) ;
#10301=FILL_AREA_STYLE ('',( #13515 ) ) ;
#10311=AXIS2_PLACEMENT_3D ( 'NONE', #7055, #49, #16225 ) ;
#10315=DIRECTION ( 'NONE',  ( 0.000000000000000000, -1.000000000000000000, 0.000000000000000000 ) ) ;
#10318=DIRECTION ( 'NONE',  ( -1.000000000000000000, -3.994014902950000436E-29, 0.000000000000000000 ) ) ;
#10325=CARTESIAN_POINT ( 'NONE',  ( -21.35824191589999899, -4.000000000000000000, -144.8157682190000060 ) ) ;
#10343=CIRCLE ( 'NONE', #13003, 1.000000000000000888 ) ;
#10347=CARTESIAN_POINT ( 'NONE',  ( -22.10824191591069265, -32.00000000000000000, -141.9623572383543717 ) ) ;
#10363=VERTEX_POINT ( 'NONE', #8974 ) ;
#10364=CARTESIAN_POINT ( 'NONE',  ( 29.68320006080000084, -24.50000000000000000, -149.3052959529999839 ) ) ;
#10407=ORIENTED_EDGE ( 'NONE', *, *, #9605, .T. ) ;
#10415=ORIENTED_EDGE ( 'NONE', *, *, #17078, .F. ) ;
#10419=ORIENTED_EDGE ( 'NONE', *, *, #2016, .T. ) ;
#10420=CARTESIAN_POINT ( 'NONE',  ( -21.35824191589999899, -4.000000000000000000, -144.8157682190000060 ) ) ;
#10427=VERTEX_POINT ( 'NONE', #22427 ) ;
#10472=CARTESIAN_POINT ( 'NONE',  ( -18.35824191589999899, -13.50000000000000000, -146.3157682190000060 ) ) ;
#10484=CARTESIAN_POINT ( 'NONE',  ( -20.60824191589185972, -4.000000000000000000, -149.4708568729739966 ) ) ;
#10490=CARTESIAN_POINT ( 'NONE',  ( 11.68320006080000262, -20.76179938779915446, -148.5552959529999839 ) ) ;
#10494=CARTESIAN_POINT ( 'NONE',  ( -7.816799939239999162, -1.500000000000000000, -150.0552959529999839 ) ) ;
#10510=ORIENTED_EDGE ( 'NONE', *, *, #14548, .F. ) ;
#10511=ORIENTED_EDGE ( 'NONE', *, *, #20346, .T. ) ;
#10531=AXIS2_PLACEMENT_3D ( 'NONE', #21432, #19409, #6781 ) ;
#10536=ORIENTED_EDGE ( 'NONE', *, *, #14317, .F. ) ;
#10546=VERTEX_POINT ( 'NONE', #15516 ) ;
#10555=ORIENTED_EDGE ( 'NONE', *, *, #21836, .F. ) ;
#10559=CARTESIAN_POINT ( 'NONE',  ( -18.07392865170000107, -1.500000000000000000, -144.8157682190000060 ) ) ;
#10560=CYLINDRICAL_SURFACE ( 'NONE', #1352, 3.499999999999999556 ) ;
#10563=DIRECTION ( 'NONE',  ( 1.000000000000000000, 0.000000000000000000, 2.516505522483685870E-12 ) ) ;
#10565=CARTESIAN_POINT ( 'NONE',  ( -15.53720866509999965, -34.50000000000000000, -147.3052959529999839 ) ) ;
#10567=CARTESIAN_POINT ( 'NONE',  ( 29.68320006080000084, -32.50000000000000000, -150.0552959529999839 ) ) ;
#10572=ORIENTED_EDGE ( 'NONE', *, *, #14864, .F. ) ;
#10580=CARTESIAN_POINT ( 'NONE',  ( 19.68320006079999729, -16.50000000000000000, -149.3052959529999839 ) ) ;
#10589=AXIS2_PLACEMENT_3D ( 'NONE', #9751, #15257, #6207 ) ;
#10604=AXIS2_PLACEMENT_3D ( 'NONE', #13943, #12500, #12269 ) ;
#10605=CIRCLE ( 'NONE', #11742, 0.7500000000000006661 ) ;
#10606=ORIENTED_EDGE ( 'NONE', *, *, #679, .T. ) ;
#10623=DIRECTION ( 'NONE',  ( 0.7071067811865481278, -0.7071067811865469066, 1.776356839400246426E-12 ) ) ;
#10624=PRODUCT_CONTEXT ( 'NONE', #16784, 'mechanical' ) ;
#10654=FACE_OUTER_BOUND ( 'NONE', #12418, .T. ) ;
#10673=DIRECTION ( 'NONE',  ( 1.211690350419999855E-27, 2.765629237170000203E-27, -1.000000000000000000 ) ) ;
#10680=CIRCLE ( 'NONE', #5386, 0.7500000000000006661 ) ;
#10688=CARTESIAN_POINT ( 'NONE',  ( 10.68320006080000084, -20.50000000000000000, -148.5552959529999839 ) ) ;
#10690=CARTESIAN_POINT ( 'NONE',  ( -21.35824191589999899, -3.250000000000000000, -144.8157682190000060 ) ) ;
#10706=ADVANCED_FACE ( 'NONE', ( #10275 ), #11813, .F. ) ;
#10745=DIRECTION ( 'NONE',  ( -1.000000000000000000, -3.994014902950000436E-29, 0.000000000000000000 ) ) ;
#10759=DIRECTION ( 'NONE',  ( 1.000000000000000000, 0.000000000000000000, 2.516505522483685870E-12 ) ) ;
#10769=CYLINDRICAL_SURFACE ( 'NONE', #20515, 1.000000000000001332 ) ;
#10778=VECTOR ( 'NONE', #18936, 1000.000000000000000 ) ;
#10783=VERTEX_POINT ( 'NONE', #18129 ) ;
#10794=ORIENTED_EDGE ( 'NONE', *, *, #14548, .T. ) ;
#10811=DIRECTION ( 'NONE',  ( -1.000000000000000000, 0.000000000000000000, 0.000000000000000000 ) ) ;
#10818=CARTESIAN_POINT ( 'NONE',  ( 10.68320006080000084, -21.50000000000000000, -148.5552959529999839 ) ) ;
#10820=EDGE_LOOP ( 'NONE', ( #9163, #20116 ) ) ;
#10829=CIRCLE ( 'NONE', #18076, 9.999999999999998224 ) ;
#10843=PLANE ( 'NONE',  #2375 ) ;
#10844=DIRECTION ( 'NONE',  ( 2.507771768019999718E-12, 1.592654864209999947E-17, -1.000000000000000000 ) ) ;
#10856=CARTESIAN_POINT ( 'NONE',  ( 19.68320006079999729, -20.50000000000000000, -150.0552959529999839 ) ) ;
#10863=EDGE_CURVE ( 'NONE', #22307, #3022, #13828, .T. ) ;
#10872=CARTESIAN_POINT ( 'NONE',  ( 29.68320006080000084, -28.50000000000000000, -150.0552959529999839 ) ) ;
#10880=CARTESIAN_POINT ( 'NONE',  ( -25.85824191589999899, -13.50000000000000000, -146.3157682190000060 ) ) ;
#10881=VERTEX_POINT ( 'NONE', #1105 ) ;
#10902=VERTEX_POINT ( 'NONE', #21654 ) ;
#10905=DIRECTION ( 'NONE',  ( -3.994014902950000436E-29, 1.000000000000000000, -4.148443855749999753E-27 ) ) ;
#10912=AXIS2_PLACEMENT_3D ( 'NONE', #19874, #4033, #23435 ) ;
#10916=LINE ( 'NONE', #3325, #8542 ) ;
#10930=PRODUCT_DEFINITION ( 'UNKNOWN', '', #22938, #16585 ) ;
#10960=EDGE_LOOP ( 'NONE', ( #9084, #8489, #13276, #16662 ) ) ;
#10982=DIRECTION ( 'NONE',  ( 1.211690350419999855E-27, 2.765629237170000203E-27, -1.000000000000000000 ) ) ;
#10986=VECTOR ( 'NONE', #6455, 1000.000000000000000 ) ;
#10994=AXIS2_PLACEMENT_3D ( 'NONE', #13433, #13197, #16776 ) ;
#11014=CIRCLE ( 'NONE', #23191, 0.7500000000000006661 ) ;
#11018=VERTEX_POINT ( 'NONE', #17097 ) ;
#11033=CARTESIAN_POINT ( 'NONE',  ( 9.183200060760000838, 0.4999999999990000776, -148.5552959529999839 ) ) ;
#11035=ADVANCED_FACE ( 'NONE', ( #334 ), #458, .T. ) ;
#11049=FACE_OUTER_BOUND ( 'NONE', #8837, .T. ) ;
#11050=CARTESIAN_POINT ( 'NONE',  ( 27.18320006080000084, 0.9999999999989999111, -150.0552959529999839 ) ) ;
#11051=DIRECTION ( 'NONE',  ( 1.000000000000000000, 0.000000000000000000, 2.516505522483685870E-12 ) ) ;
#11064=EDGE_CURVE ( 'NONE', #19530, #18104, #16977, .T. ) ;
#11074=AXIS2_PLACEMENT_3D ( 'NONE', #14088, #10844, #8944 ) ;
#11077=DIRECTION ( 'NONE',  ( 1.000000000000000000, 0.000000000000000000, 0.000000000000000000 ) ) ;
#11089=VERTEX_POINT ( 'NONE', #2369 ) ;
#11094=CARTESIAN_POINT ( 'NONE',  ( 10.68320006080000084, -20.50000000000000000, -150.0552959529999839 ) ) ;
#11103=STYLED_ITEM ( 'NONE', ( #541 ), #10046 ) ;
#11105=VECTOR ( 'NONE', #6215, 1000.000000000000000 ) ;
#11108=EDGE_CURVE ( 'NONE', #17890, #6188, #12085, .T. ) ;
#11116=EDGE_CURVE ( 'NONE', #19064, #17007, #11846, .T. ) ;
#11140=VERTEX_POINT ( 'NONE', #21626 ) ;
#11145=DIRECTION ( 'NONE',  ( 0.000000000000000000, -4.148443855749999753E-27, -1.000000000000000000 ) ) ;
#11151=DIRECTION ( 'NONE',  ( 1.211690350419999855E-27, 2.765629237170000203E-27, -1.000000000000000000 ) ) ;
#11163=CARTESIAN_POINT ( 'NONE',  ( -21.35824191589999899, -32.00000000000000000, -146.2257682199999920 ) ) ;
#11166=EDGE_CURVE ( 'NONE', #22352, #3173, #194, .T. ) ;
#11173=CARTESIAN_POINT ( 'NONE',  ( -21.74973190997082284, -4.669170177705934677, -146.3157682190010007 ) ) ;
#11185=DIRECTION ( 'NONE',  ( -0.9848077530125619594, 0.000000000000000000, -0.1736481776649230202 ) ) ;
#11193=CARTESIAN_POINT ( 'NONE',  ( 9.709183429561321077, -20.23902802861211114, -148.5552959530000123 ) ) ;
#11195=DIRECTION ( 'NONE',  ( 0.000000000000000000, 0.000000000000000000, 1.000000000000000000 ) ) ;
#11202=VECTOR ( 'NONE', #17618, 1000.000000000000227 ) ;
#11213=DIRECTION ( 'NONE',  ( -2.507771768022264771E-12, -1.592655090489709912E-17, 1.000000000000000000 ) ) ;
#11225=LINE ( 'NONE', #16486, #17806 ) ;
#11232=VECTOR ( 'NONE', #9547, 1000.000000000000000 ) ;
#11262=LINE ( 'NONE', #20227, #3309 ) ;
#11287=CARTESIAN_POINT ( 'NONE',  ( 10.81534092360039701, -19.49999999999999645, -148.5552959529999839 ) ) ;
#11291=ADVANCED_FACE ( 'NONE', ( #20886 ), #19203, .F. ) ;
#11294=CARTESIAN_POINT ( 'NONE',  ( 29.68320006080000084, -16.50000000000000000, -150.0552959529999839 ) ) ;
#11300=CARTESIAN_POINT ( 'NONE',  ( -18.07392865170000107, -34.50000000000000000, -146.3157682190000060 ) ) ;
#11305=VECTOR ( 'NONE', #6166, 1000.000000000000000 ) ;
#11322=CARTESIAN_POINT ( 'NONE',  ( -25.35824191590000254, -18.00000000000000000, -146.3157682190000060 ) ) ;
#11336=AXIS2_PLACEMENT_3D ( 'NONE', #18794, #2279, #16773 ) ;
#11343=ADVANCED_FACE ( 'NONE', ( #1145 ), #11695, .F. ) ;
#11345=EDGE_CURVE ( 'NONE', #5391, #16441, #3041, .T. ) ;
#11355=ORIENTED_EDGE ( 'NONE', *, *, #13026, .F. ) ;
#11362=B_SPLINE_CURVE_WITH_KNOTS ( 'NONE', 3,
 ( #10818, #1700, #1938, #17989, #16318, #12974, #1813, #3702, #14414, #1587 ),
 .UNSPECIFIED., .F., .F.,
 ( 4, 2, 2, 2, 4 ),
 ( 0.000000000000000000, 0.2500000000000000000, 0.5000000000000000000, 0.7500000000000000000, 1.000000000000000000 ),
 .UNSPECIFIED. ) ;
#11368=CARTESIAN_POINT ( 'NONE',  ( -25.35824191590000254, -1.500000000000000000, -145.5657682199999954 ) ) ;
#11377=CIRCLE ( 'NONE', #18254, 10.00000000000000000 ) ;
#11379=CARTESIAN_POINT ( 'NONE',  ( -14.47770030809999930, -15.50000000000000000, -147.5552959529999839 ) ) ;
#11381=FACE_OUTER_BOUND ( 'NONE', #4842, .T. ) ;
#11382=ORIENTED_EDGE ( 'NONE', *, *, #12997, .T. ) ;
#11390=AXIS2_PLACEMENT_3D ( 'NONE', #20554, #11719, #19001 ) ;
#11391=AXIS2_PLACEMENT_3D ( 'NONE', #814, #7580, #9350 ) ;
#11392=ORIENTED_EDGE ( 'NONE', *, *, #13153, .F. ) ;
#11393=CARTESIAN_POINT ( 'NONE',  ( -26.35824191589999899, -1.500000000000000000, -141.0657682190000060 ) ) ;
#11407=ADVANCED_FACE ( 'NONE', ( #20038 ), #5054, .T. ) ;
#11436=ORIENTED_EDGE ( 'NONE', *, *, #5963, .T. ) ;
#11440=DIRECTION ( 'NONE',  ( 3.994014902950000436E-29, -1.000000000000000000, 4.148443855749999753E-27 ) ) ;
#11447=B_SPLINE_CURVE_WITH_KNOTS ( 'NONE', 3,
 ( #16417, #12830, #17846, #7472, #5223, #7253, #18081, #14273 ),
 .UNSPECIFIED., .F., .F.,
 ( 4, 2, 2, 4 ),
 ( 0.000000000000000000, 0.5000000000000031086, 0.7500000000000015543, 1.000000000000000000 ),
 .UNSPECIFIED. ) ;
#11465=CARTESIAN_POINT ( 'NONE',  ( -18.35824191589999899, -34.50000000000000000, -150.0657682190000060 ) ) ;
#11470=DIRECTION ( 'NONE',  ( 1.000000000000000000, 0.000000000000000000, 2.516505522483685870E-12 ) ) ;
#11476=ORIENTED_EDGE ( 'NONE', *, *, #18776, .F. ) ;
#11484=ADVANCED_FACE ( 'NONE', ( #1965 ), #7180, .T. ) ;
#11487=DIRECTION ( 'NONE',  ( 2.508215857230000030E-12, 0.000000000000000000, -1.000000000000000000 ) ) ;
#11524=ORIENTED_EDGE ( 'NONE', *, *, #19945, .T. ) ;
#11525=ORIENTED_EDGE ( 'NONE', *, *, #22979, .F. ) ;
#11531=ORIENTED_EDGE ( 'NONE', *, *, #22917, .F. ) ;
#11532=CARTESIAN_POINT ( 'NONE',  ( -16.20111387579999729, -34.50000000000000000, -147.8591802640000026 ) ) ;
#11549=ORIENTED_EDGE ( 'NONE', *, *, #9872, .T. ) ;
#11598=B_SPLINE_CURVE_WITH_KNOTS ( 'NONE', 3,
 ( #22023, #9619, #11173, #20357, #603, #20589 ),
 .UNSPECIFIED., .F., .F.,
 ( 4, 2, 4 ),
 ( 0.000000000000000000, 0.5000000000000000000, 1.000000000000000000 ),
 .UNSPECIFIED. ) ;
#11609=EDGE_CURVE ( 'NONE', #15560, #22352, #1209, .T. ) ;
#11660=ADVANCED_FACE ( 'NONE', ( #4428 ), #17159, .F. ) ;
#11666=DIRECTION ( 'NONE',  ( 1.000000000000000000, 0.000000000000000000, 0.000000000000000000 ) ) ;
#11691=DIRECTION ( 'NONE',  ( 1.000000000000000000, 0.000000000000000000, 0.000000000000000000 ) ) ;
#11695=CYLINDRICAL_SURFACE ( 'NONE', #11784, 0.7500000000000006661 ) ;
#11702=FACE_OUTER_BOUND ( 'NONE', #11953, .T. ) ;
#11706=CARTESIAN_POINT ( 'NONE',  ( 9.183200060760000838, 0.4999999999990000776, -148.5552959529999839 ) ) ;
#11707=EDGE_CURVE ( 'NONE', #11140, #2330, #20550, .T. ) ;
#11712=VECTOR ( 'NONE', #5245, 1000.000000000000000 ) ;
#11717=ORIENTED_EDGE ( 'NONE', *, *, #10102, .F. ) ;
#11719=DIRECTION ( 'NONE',  ( -2.507771768022264771E-12, -1.592655090489709912E-17, 1.000000000000000000 ) ) ;
#11725=ORIENTED_EDGE ( 'NONE', *, *, #5620, .T. ) ;
#11733=CARTESIAN_POINT ( 'NONE',  ( -25.85824191589999899, -34.50000000000000000, -144.8157682190000060 ) ) ;
#11736=VECTOR ( 'NONE', #19070, 1000.000000000000000 ) ;
#11742=AXIS2_PLACEMENT_3D ( 'NONE', #20142, #6083, #9167 ) ;
#11749=AXIS2_PLACEMENT_3D ( 'NONE', #11050, #18328, #2040 ) ;
#11758=VERTEX_POINT ( 'NONE', #10484 ) ;
#11765=DIRECTION ( 'NONE',  ( -1.211690350419999855E-27, -2.765629237170000203E-27, 1.000000000000000000 ) ) ;
#11773=CARTESIAN_POINT ( 'NONE',  ( 19.68320006079999729, -16.50000000000000000, -150.0552959529999839 ) ) ;
#11784=AXIS2_PLACEMENT_3D ( 'NONE', #15403, #4814, #15646 ) ;
#11804=ORIENTED_EDGE ( 'NONE', *, *, #22047, .F. ) ;
#11811=DIRECTION ( 'NONE',  ( 1.211690350419999855E-27, 2.765629237170000203E-27, -1.000000000000000000 ) ) ;
#11813=PLANE ( 'NONE',  #8727 ) ;
#11823=DIRECTION ( 'NONE',  ( 1.211690350419999855E-27, 2.765629237170000203E-27, -1.000000000000000000 ) ) ;
#11835=ORIENTED_EDGE ( 'NONE', *, *, #5736, .F. ) ;
#11846=LINE ( 'NONE', #15783, #2326 ) ;
#11849=ADVANCED_FACE ( 'NONE', ( #7294 ), #3724, .T. ) ;
#11853=VECTOR ( 'NONE', #7491, 1000.000000000000000 ) ;
#11863=DIRECTION ( 'NONE',  ( -2.808280234689999718E-18, 1.000000000000000000, 1.592654863659999653E-17 ) ) ;
#11864=DIRECTION ( 'NONE',  ( 0.000000000000000000, 0.000000000000000000, 1.000000000000000000 ) ) ;
#11865=EDGE_CURVE ( 'NONE', #1186, #6741, #23243, .T. ) ;
#11866=ORIENTED_EDGE ( 'NONE', *, *, #13457, .T. ) ;
#11867=FACE_OUTER_BOUND ( 'NONE', #22528, .T. ) ;
#11872=ORIENTED_EDGE ( 'NONE', *, *, #6702, .T. ) ;
#11878=ORIENTED_EDGE ( 'NONE', *, *, #11865, .F. ) ;
#11886=DIRECTION ( 'NONE',  ( -3.994014904670000134E-29, 1.000000000000000000, 0.000000000000000000 ) ) ;
#11890=LINE ( 'NONE', #6423, #7126 ) ;
#11897=LINE ( 'NONE', #19165, #441 ) ;
#11903=CARTESIAN_POINT ( 'NONE',  ( 27.68320006080000084, -32.50000000000000000, -148.5552959529999839 ) ) ;
#11924=EDGE_CURVE ( 'NONE', #10881, #8290, #13679, .T. ) ;
#11948=ORIENTED_EDGE ( 'NONE', *, *, #16204, .T. ) ;
#11953=EDGE_LOOP ( 'NONE', ( #2563, #14849 ) ) ;
#11957=CIRCLE ( 'NONE', #19977, 2.500000000000000444 ) ;
#11959=VERTEX_POINT ( 'NONE', #18816 ) ;
#11961=CARTESIAN_POINT ( 'NONE',  ( -25.85824191589999899, -34.50000000000000000, -146.3157682190000060 ) ) ;
#11964=CARTESIAN_POINT ( 'NONE',  ( -20.60824191589999899, -4.000000000000000000, -141.0657682190000060 ) ) ;
#11968=ORIENTED_EDGE ( 'NONE', *, *, #9382, .F. ) ;
#11993=AXIS2_PLACEMENT_3D ( 'NONE', #18057, #1771, #21872 ) ;
#11998=ORIENTED_EDGE ( 'NONE', *, *, #5882, .F. ) ;
#12001=ADVANCED_FACE ( 'NONE', ( #8095 ), #17625, .T. ) ;
#12017=CYLINDRICAL_SURFACE ( 'NONE', #77, 0.7500000000000006661 ) ;
#12019=ORIENTED_EDGE ( 'NONE', *, *, #22589, .F. ) ;
#12024=VERTEX_POINT ( 'NONE', #10108 ) ;
#12050=PLANE ( 'NONE',  #3500 ) ;
#12051=CARTESIAN_POINT ( 'NONE',  ( 11.57542696440981089, -21.02198665876327510, -148.5552959529999839 ) ) ;
#12055=PLANE ( 'NONE',  #7219 ) ;
#12058=CIRCLE ( 'NONE', #4084, 2.500000000000000000 ) ;
#12085=LINE ( 'NONE', #17212, #13702 ) ;
#12098=CARTESIAN_POINT ( 'NONE',  ( -21.35824191589999899, -4.750000000000000000, -146.3157682190075093 ) ) ;
#12101=CYLINDRICAL_SURFACE ( 'NONE', #20521, 1.000000000000004219 ) ;
#12117=FACE_OUTER_BOUND ( 'NONE', #23183, .T. ) ;
#12151=AXIS2_PLACEMENT_3D ( 'NONE', #10856, #14679, #18261 ) ;
#12174=FACE_OUTER_BOUND ( 'NONE', #17657, .T. ) ;
#12178=FACE_OUTER_BOUND ( 'NONE', #4829, .T. ) ;
#12180=ORIENTED_EDGE ( 'NONE', *, *, #12992, .T. ) ;
#12185=AXIS2_PLACEMENT_3D ( 'NONE', #9761, #13466, #11666 ) ;
#12186=CARTESIAN_POINT ( 'NONE',  ( -18.07392865170000107, -1.500000000000000000, -146.3157682190000060 ) ) ;
#12190=EDGE_CURVE ( 'NONE', #4104, #16441, #22468, .T. ) ;
#12213=CARTESIAN_POINT ( 'NONE',  ( -21.35824191589999899, -4.750000000000000000, -144.8157682190000060 ) ) ;
#12214=VECTOR ( 'NONE', #5117, 1000.000000000000000 ) ;
#12219=DIRECTION ( 'NONE',  ( 1.000000000000000000, 0.000000000000000000, 2.516505522483685870E-12 ) ) ;
#12233=ORIENTED_EDGE ( 'NONE', *, *, #22879, .T. ) ;
#12245=EDGE_LOOP ( 'NONE', ( #15154, #11725, #13445, #12569 ) ) ;
#12248=ADVANCED_FACE ( 'NONE', ( #16770 ), #7948, .F. ) ;
#12257=LINE ( 'NONE', #21911, #17888 ) ;
#12263=ORIENTED_EDGE ( 'NONE', *, *, #14108, .T. ) ;
#12269=DIRECTION ( 'NONE',  ( 0.000000000000000000, -4.148443855749999753E-27, -1.000000000000000000 ) ) ;
#12276=VERTEX_POINT ( 'NONE', #15668 ) ;
#12286=EDGE_LOOP ( 'NONE', ( #7299, #23384, #21689, #200 ) ) ;
#12295=DIRECTION ( 'NONE',  ( -0.1736481776649230480, 0.000000000000000000, 0.9848077530125620704 ) ) ;
#12304=CYLINDRICAL_SURFACE ( 'NONE', #20042, 0.7500000000000016653 ) ;
#12310=ORIENTED_EDGE ( 'NONE', *, *, #14112, .T. ) ;
#12316=VECTOR ( 'NONE', #14907, 1000.000000000000000 ) ;
#12334=DIRECTION ( 'NONE',  ( -1.211690350419999855E-27, -2.765629237170000203E-27, 1.000000000000000000 ) ) ;
#12343=DIRECTION ( 'NONE',  ( 1.000000000000000000, 0.000000000000000000, 0.000000000000000000 ) ) ;
#12361=DIRECTION ( 'NONE',  ( 0.000000000000000000, 1.000000000000000000, 0.000000000000000000 ) ) ;
#12370=DIRECTION ( 'NONE',  ( 1.000000000000000000, 0.000000000000000000, 2.516505522483685870E-12 ) ) ;
#12371=CARTESIAN_POINT ( 'NONE',  ( -15.53720866509999965, -1.500000000000000000, -147.3052959529999839 ) ) ;
#12391=ORIENTED_EDGE ( 'NONE', *, *, #23052, .T. ) ;
#12403=ORIENTED_EDGE ( 'NONE', *, *, #14784, .T. ) ;
#12409=CARTESIAN_POINT ( 'NONE',  ( -16.93971969060000049, -34.50000000000000000, -147.9894163970000136 ) ) ;
#12418=EDGE_LOOP ( 'NONE', ( #6646, #11948, #9555, #19327 ) ) ;
#12441=CARTESIAN_POINT ( 'NONE',  ( 11.68320006079999906, -20.50000000000000000, -148.5552959529999839 ) ) ;
#12445=CIRCLE ( 'NONE', #13971, 25.00000000000000000 ) ;
#12455=ADVANCED_FACE ( 'NONE', ( #22050 ), #10843, .F. ) ;
#12469=DIRECTION ( 'NONE',  ( 0.000000000000000000, 0.000000000000000000, 1.000000000000000000 ) ) ;
#12481=CARTESIAN_POINT ( 'NONE',  ( 27.68320006080000084, -32.50000000000000000, -150.0552959529999839 ) ) ;
#12487=CIRCLE ( 'NONE', #1117, 1.000000000000000888 ) ;
#12488=DIRECTION ( 'NONE',  ( 2.507554887169999917E-12, 0.000000000000000000, -1.000000000000000000 ) ) ;
#12489=VECTOR ( 'NONE', #13405, 1000.000000000000000 ) ;
#12490=DIRECTION ( 'NONE',  ( 0.000000000000000000, 1.000000000000000000, 0.000000000000000000 ) ) ;
#12500=DIRECTION ( 'NONE',  ( -3.994014902950000436E-29, 1.000000000000000000, -4.148443855749999753E-27 ) ) ;
#12523=ORIENTED_EDGE ( 'NONE', *, *, #20595, .F. ) ;
#12534=SHAPE_DEFINITION_REPRESENTATION ( #7390, #23186 ) ;
#12535=FACE_OUTER_BOUND ( 'NONE', #19215, .T. ) ;
#12557=VECTOR ( 'NONE', #6241, 1000.000000000000000 ) ;
#12569=ORIENTED_EDGE ( 'NONE', *, *, #21321, .F. ) ;
#12573=AXIS2_PLACEMENT_3D ( 'NONE', #13580, #17395, #8342 ) ;
#12578=LINE ( 'NONE', #14609, #6410 ) ;
#12582=EDGE_LOOP ( 'NONE', ( #12523, #5971, #17134, #4250 ) ) ;
#12586=EDGE_LOOP ( 'NONE', ( #11968, #5991, #15135, #21141 ) ) ;
#12601=DIRECTION ( 'NONE',  ( -1.000000000000000000, -3.717264591378872697E-16, 0.000000000000000000 ) ) ;
#12608=CARTESIAN_POINT ( 'NONE',  ( -18.07392865170000107, -18.00000000000000000, -146.3157682190000060 ) ) ;
#12624=EDGE_CURVE ( 'NONE', #6697, #11089, #15132, .T. ) ;
#12633=ORIENTED_EDGE ( 'NONE', *, *, #20027, .F. ) ;
#12637=DIRECTION ( 'NONE',  ( -2.507771768023035002E-12, -1.592654560756634986E-17, 1.000000000000000000 ) ) ;
#12648=CARTESIAN_POINT ( 'NONE',  ( 18.18320006080000084, -6.500000000000000000, -148.5552959529999839 ) ) ;
#12673=ORIENTED_EDGE ( 'NONE', *, *, #22202, .T. ) ;
#12677=DIRECTION ( 'NONE',  ( 0.000000000000000000, 1.000000000000000000, 0.000000000000000000 ) ) ;
#12706=DIRECTION ( 'NONE',  ( -2.507771768019999718E-12, 0.000000000000000000, 1.000000000000000000 ) ) ;
#12712=LINE ( 'NONE', #6891, #20787 ) ;
#12714=ADVANCED_FACE ( 'NONE', ( #7978 ), #22515, .F. ) ;
#12722=LINE ( 'NONE', #3222, #12968 ) ;
#12734=VERTEX_POINT ( 'NONE', #14056 ) ;
#12735=LINE ( 'NONE', #7149, #11712 ) ;
#12762=AXIS2_PLACEMENT_3D ( 'NONE', #9018, #21547, #23440 ) ;
#12780=SURFACE_SIDE_STYLE ('',( #420 ) ) ;
#12800=ORIENTED_EDGE ( 'NONE', *, *, #13969, .T. ) ;
#12802=CARTESIAN_POINT ( 'NONE',  ( 27.18320006080000084, 3.500000000000000000, -148.5552959529999839 ) ) ;
#12803=AXIS2_PLACEMENT_3D ( 'NONE', #1974, #10982, #22291 ) ;
#12818=DIRECTION ( 'NONE',  ( 1.211690350419999855E-27, 2.765629237170000203E-27, -1.000000000000000000 ) ) ;
#12821=CARTESIAN_POINT ( 'NONE',  ( -18.35824191589999899, -34.50000000000000000, -144.8157682190000060 ) ) ;
#12830=CARTESIAN_POINT ( 'NONE',  ( -21.16045305574322200, -4.749999999999998224, -146.3157682190070830 ) ) ;
#12860=DIRECTION ( 'NONE',  ( 3.994014902950000436E-29, -1.000000000000000000, 4.148443855749999753E-27 ) ) ;
#12866=CARTESIAN_POINT ( 'NONE',  ( 25.18320006080000084, -34.50000000000000000, -148.5552959529999839 ) ) ;
#12868=VECTOR ( 'NONE', #19150, 1000.000000000000000 ) ;
#12917=AXIS2_PLACEMENT_3D ( 'NONE', #17957, #10673, #23425 ) ;
#12935=LINE ( 'NONE', #7574, #16326 ) ;
#12947=VECTOR ( 'NONE', #4850, 1000.000000000000000 ) ;
#12954=ORIENTED_EDGE ( 'NONE', *, *, #3277, .F. ) ;
#12968=VECTOR ( 'NONE', #6901, 1000.000000000000000 ) ;
#12973=EDGE_CURVE ( 'NONE', #10427, #1513, #14756, .T. ) ;
#12974=CARTESIAN_POINT ( 'NONE',  ( 9.882881882281347785, -21.11395234859968184, -148.5552959529999839 ) ) ;
#12985=AXIS2_PLACEMENT_3D ( 'NONE', #3606, #7401, #8937 ) ;
#12989=FACE_OUTER_BOUND ( 'NONE', #16375, .T. ) ;
#12992=EDGE_CURVE ( 'NONE', #3932, #10783, #2507, .T. ) ;
#12994=DIRECTION ( 'NONE',  ( -2.507771768019999718E-12, -1.592654864069999939E-17, 1.000000000000000000 ) ) ;
#12997=EDGE_CURVE ( 'NONE', #15090, #10047, #6925, .T. ) ;
#13003=AXIS2_PLACEMENT_3D ( 'NONE', #6758, #2621, #953 ) ;
#13013=CARTESIAN_POINT ( 'NONE',  ( -18.07392865170000107, -34.50000000000000000, -147.3157682190000060 ) ) ;
#13019=CIRCLE ( 'NONE', #9590, 1.000000000000000888 ) ;
#13026=EDGE_CURVE ( 'NONE', #11018, #16936, #18445, .T. ) ;
#13035=ADVANCED_FACE ( 'NONE', ( #15105 ), #5825, .F. ) ;
#13041=CARTESIAN_POINT ( 'NONE',  ( 10.93320006080000084, 3.500000000000000000, -150.0552959529999839 ) ) ;
#13057=LINE ( 'NONE', #4021, #19089 ) ;
#13059=DIRECTION ( 'NONE',  ( 1.000000000000000000, 0.000000000000000000, 0.000000000000000000 ) ) ;
#13062=CARTESIAN_POINT ( 'NONE',  ( -21.35824191589999899, -32.00000000000000000, -141.0657682190000060 ) ) ;
#13068=DIRECTION ( 'NONE',  ( -1.211690350419999855E-27, -2.765629237170000203E-27, 1.000000000000000000 ) ) ;
#13073=ORIENTED_EDGE ( 'NONE', *, *, #279, .F. ) ;
#13076=DIRECTION ( 'NONE',  ( -2.507771768019999718E-12, -1.592654864069999939E-17, 1.000000000000000000 ) ) ;
#13083=CARTESIAN_POINT ( 'NONE',  ( -21.35824191589999899, -4.000000000000000000, -144.8157682190000060 ) ) ;
#13087=VECTOR ( 'NONE', #14538, 1000.000000000000000 ) ;
#13114=ORIENTED_CLOSED_SHELL ( 'NONE', *, #6122, .F. );
#13121=LINE ( 'NONE', #11322, #11232 ) ;
#13128=EDGE_LOOP ( 'NONE', ( #18917, #2608, #4696, #19829 ) ) ;
#13153=EDGE_CURVE ( 'NONE', #15515, #1286, #10343, .T. ) ;
#13172=CARTESIAN_POINT ( 'NONE',  ( -18.35824191589999899, -18.00000000000000000, -150.0657682190000060 ) ) ;
#13181=VECTOR ( 'NONE', #11185, 1000.000000000000227 ) ;
#13197=DIRECTION ( 'NONE',  ( 2.507771768019999718E-12, 1.592654864209999947E-17, -1.000000000000000000 ) ) ;
#13205=CARTESIAN_POINT ( 'NONE',  ( -21.35824191589999899, -4.000000000000000000, -146.2257682199999920 ) ) ;
#13207=CARTESIAN_POINT ( 'NONE',  ( -21.35824191589999899, -31.25000000000000000, -144.8157682190000060 ) ) ;
#13217=AXIS2_PLACEMENT_3D ( 'NONE', #2466, #10037, #6135 ) ;
#13222=CARTESIAN_POINT ( 'NONE',  ( -18.07392865170000107, -18.00000000000000000, -144.8157682190000060 ) ) ;
#13235=ADVANCED_FACE ( 'NONE', ( #19859 ), #5457, .T. ) ;
#13241=CARTESIAN_POINT ( 'NONE',  ( 29.68320006080000084, 0.9999999999989999111, -150.0552959529999839 ) ) ;
#13246=CIRCLE ( 'NONE', #2269, 2.500000000000000444 ) ;
#13250=LINE ( 'NONE', #13373, #18393 ) ;
#13251=CIRCLE ( 'NONE', #1509, 0.7500000000000006661 ) ;
#13265=CIRCLE ( 'NONE', #6433, 9.999999999999998224 ) ;
#13271=ORIENTED_EDGE ( 'NONE', *, *, #8938, .T. ) ;
#13276=ORIENTED_EDGE ( 'NONE', *, *, #19570, .F. ) ;
#13291=FACE_OUTER_BOUND ( 'NONE', #23309, .T. ) ;
#13295=EDGE_LOOP ( 'NONE', ( #15428, #4630, #5674, #13845 ) ) ;
#13304=VECTOR ( 'NONE', #13059, 1000.000000000000000 ) ;
#13305=ORIENTED_EDGE ( 'NONE', *, *, #19917, .T. ) ;
#13306=PLANE ( 'NONE',  #5685 ) ;
#13308=ORIENTED_EDGE ( 'NONE', *, *, #676, .F. ) ;
#13315=CARTESIAN_POINT ( 'NONE',  ( -18.07392865170000107, -34.50000000000000000, -145.5657682190000060 ) ) ;
#13322=CARTESIAN_POINT ( 'NONE',  ( -21.35824191591069265, -32.00000000000000000, -141.9623572383524959 ) ) ;
#13327=ADVANCED_FACE ( 'NONE', ( #1552 ), #16168, .F. ) ;
#13333=EDGE_LOOP ( 'NONE', ( #23510, #7817, #6520, #7645 ) ) ;
#13339=AXIS2_PLACEMENT_3D ( 'NONE', #4734, #8164, #17222 ) ;
#13347=ORIENTED_EDGE ( 'NONE', *, *, #2409, .T. ) ;
#13362=LINE ( 'NONE', #4327, #5965 ) ;
#13366=ORIENTED_EDGE ( 'NONE', *, *, #16819, .T. ) ;
#13368=ORIENTED_EDGE ( 'NONE', *, *, #11924, .T. ) ;
#13373=CARTESIAN_POINT ( 'NONE',  ( 24.68320006080000084, -24.50000000000000000, -150.0552959529999839 ) ) ;
#13405=DIRECTION ( 'NONE',  ( -1.000000000000000000, 0.000000000000000000, -2.508215857230000030E-12 ) ) ;
#13406=EDGE_LOOP ( 'NONE', ( #23280, #13533, #16200, #8398 ) ) ;
#13411=ORIENTED_EDGE ( 'NONE', *, *, #10863, .T. ) ;
#13418=ADVANCED_FACE ( 'NONE', ( #6028 ), #16743, .T. ) ;
#13433=CARTESIAN_POINT ( 'NONE',  ( -21.35824191589999899, -32.00000000000000000, -146.3157682190000060 ) ) ;
#13445=ORIENTED_EDGE ( 'NONE', *, *, #22979, .T. ) ;
#13453=CARTESIAN_POINT ( 'NONE',  ( 10.06924771219168235, -19.69968182150093128, -148.5552959529999839 ) ) ;
#13457=EDGE_CURVE ( 'NONE', #11758, #22236, #13057, .T. ) ;
#13466=DIRECTION ( 'NONE',  ( -1.211690350419999855E-27, -2.765629237170000203E-27, 1.000000000000000000 ) ) ;
#13478=EDGE_CURVE ( 'NONE', #7389, #17215, #4605, .T. ) ;
#13483=ADVANCED_FACE ( 'NONE', ( #4838 ), #10050, .T. ) ;
#13489=AXIS2_PLACEMENT_3D ( 'NONE', #11294, #18921, #20710 ) ;
#13510=ORIENTED_EDGE ( 'NONE', *, *, #4952, .T. ) ;
#13513=DIRECTION ( 'NONE',  ( 0.000000000000000000, 1.000000000000000000, 0.000000000000000000 ) ) ;
#13515=FILL_AREA_STYLE_COLOUR ( '', #7419 ) ;
#13517=B_SPLINE_CURVE_WITH_KNOTS ( 'NONE', 3,
 ( #1044, #2713, #15425, #1292, #2942, #13880 ),
 .UNSPECIFIED., .F., .F.,
 ( 4, 2, 4 ),
 ( 0.000000000000000000, 0.5000000000000000000, 1.000000000000000000 ),
 .UNSPECIFIED. ) ;
#13519=ORIENTED_EDGE ( 'NONE', *, *, #3474, .T. ) ;
#13523=CARTESIAN_POINT ( 'NONE',  ( 27.18320006080000084, 0.9999999999989999111, -150.0552959529999839 ) ) ;
#13533=ORIENTED_EDGE ( 'NONE', *, *, #6555, .F. ) ;
#13539=VECTOR ( 'NONE', #20828, 1000.000000000000000 ) ;
#13552=ORIENTED_EDGE ( 'NONE', *, *, #5882, .T. ) ;
#13574=ORIENTED_EDGE ( 'NONE', *, *, #8809, .F. ) ;
#13580=CARTESIAN_POINT ( 'NONE',  ( -14.47770030809999930, -1.500000000000000000, -147.5552959529999839 ) ) ;
#13583=CARTESIAN_POINT ( 'NONE',  ( 11.53320006080000049, -24.50000000000000000, -148.5552959529999839 ) ) ;
#13600=EDGE_LOOP ( 'NONE', ( #6276, #20778, #8567, #10064 ) ) ;
#13638=DIRECTION ( 'NONE',  ( -2.508215857230000030E-12, 0.000000000000000000, 1.000000000000000000 ) ) ;
#13658=DIRECTION ( 'NONE',  ( -2.507771768019999718E-12, 0.000000000000000000, 1.000000000000000000 ) ) ;
#13668=AXIS2_PLACEMENT_3D ( 'NONE', #1330, #8907, #6900 ) ;
#13674=EDGE_CURVE ( 'NONE', #7230, #23083, #14910, .T. ) ;
#13679=B_SPLINE_CURVE_WITH_KNOTS ( 'NONE', 3,
 ( #18712, #270, #11193, #15256, #5735, #13453, #9289, #16679, #20266, #4415 ),
 .UNSPECIFIED., .F., .F.,
 ( 4, 2, 2, 2, 4 ),
 ( 0.000000000000000000, 0.2500000000000000000, 0.5000000000000000000, 0.7500000000000000000, 1.000000000000000000 ),
 .UNSPECIFIED. ) ;
#13701=VECTOR ( 'NONE', #10811, 1000.000000000000000 ) ;
#13702=VECTOR ( 'NONE', #13638, 1000.000000000000000 ) ;
#13724=ORIENTED_EDGE ( 'NONE', *, *, #3592, .F. ) ;
#13726=( NAMED_UNIT ( * ) SI_UNIT ( $, .STERADIAN. ) SOLID_ANGLE_UNIT ( ) );
#13737=VECTOR ( 'NONE', #43, 1000.000000000000000 ) ;
#13760=VERTEX_POINT ( 'NONE', #10000 ) ;
#13788=DIRECTION ( 'NONE',  ( -3.994014902717275590E-29, 1.000000000000000000, -4.148443855747225317E-27 ) ) ;
#13806=ORIENTED_EDGE ( 'NONE', *, *, #768, .F. ) ;
#13808=ORIENTED_EDGE ( 'NONE', *, *, #2589, .F. ) ;
#13818=DIRECTION ( 'NONE',  ( 0.000000000000000000, 1.000000000000000000, 0.000000000000000000 ) ) ;
#13821=ORIENTED_EDGE ( 'NONE', *, *, #22193, .F. ) ;
#13828=LINE ( 'NONE', #6214, #16721 ) ;
#13845=ORIENTED_EDGE ( 'NONE', *, *, #15215, .T. ) ;
#13880=CARTESIAN_POINT ( 'NONE',  ( -21.35824191589811605, -3.250000000000000000, -146.3157682190075093 ) ) ;
#13892=EDGE_CURVE ( 'NONE', #17215, #8780, #13019, .T. ) ;
#13911=EDGE_CURVE ( 'NONE', #1861, #10881, #11362, .T. ) ;
#13923=LINE ( 'NONE', #4880, #16259 ) ;
#13927=CARTESIAN_POINT ( 'NONE',  ( -20.60824191589999899, -32.00000000000000000, -146.2257682199999920 ) ) ;
#13943=CARTESIAN_POINT ( 'NONE',  ( 29.68320006080000084, -24.50000000000000000, -150.0552959529999839 ) ) ;
#13963=LINE ( 'NONE', #4692, #5105 ) ;
#13969=EDGE_CURVE ( 'NONE', #7704, #10902, #12735, .T. ) ;
#13971=AXIS2_PLACEMENT_3D ( 'NONE', #22009, #11863, #17111 ) ;
#14056=CARTESIAN_POINT ( 'NONE',  ( 19.68320006079999729, -16.50000000000000000, -148.5552959529999839 ) ) ;
#14088=CARTESIAN_POINT ( 'NONE',  ( -21.35824191589999899, -32.00000000000000000, -146.3157682190000060 ) ) ;
#14089=CARTESIAN_POINT ( 'NONE',  ( 11.20518671956328483, -21.39222690360982426, -148.5552959530000123 ) ) ;
#14108=EDGE_CURVE ( 'NONE', #8290, #6185, #2880, .T. ) ;
#14112=EDGE_CURVE ( 'NONE', #20629, #1, #1494, .T. ) ;
#14113=ORIENTED_EDGE ( 'NONE', *, *, #3364, .T. ) ;
#14124=ORIENTED_EDGE ( 'NONE', *, *, #15844, .T. ) ;
#14182=EDGE_LOOP ( 'NONE', ( #2467, #23030 ) ) ;
#14188=EDGE_CURVE ( 'NONE', #20598, #19064, #3207, .T. ) ;
#14191=ORIENTED_EDGE ( 'NONE', *, *, #279, .T. ) ;
#14196=FACE_OUTER_BOUND ( 'NONE', #408, .T. ) ;
#14214=CARTESIAN_POINT ( 'NONE',  ( -21.35824191589999899, -32.00000000000000000, -144.8157682190000060 ) ) ;
#14246=CARTESIAN_POINT ( 'NONE',  ( -21.35824191589999899, -4.000000000000000000, -146.2257682199999920 ) ) ;
#14248=CARTESIAN_POINT ( 'NONE',  ( -18.35824191589999899, -1.500000000000000000, -144.8157682190000060 ) ) ;
#14273=CARTESIAN_POINT ( 'NONE',  ( -20.60824191589811605, -4.000000000000000000, -146.3157682190056335 ) ) ;
#14292=ORIENTED_EDGE ( 'NONE', *, *, #1957, .F. ) ;
#14296=VECTOR ( 'NONE', #15464, 1000.000000000000000 ) ;
#14306=DIRECTION ( 'NONE',  ( 1.000000000000000000, 0.000000000000000000, 0.000000000000000000 ) ) ;
#14317=EDGE_CURVE ( 'NONE', #6977, #10222, #1429, .T. ) ;
#14332=LINE ( 'NONE', #19927, #9750 ) ;
#14336=ADVANCED_FACE ( 'NONE', ( #12117, #9973, #958 ), #2976, .T. ) ;
#14339=ORIENTED_EDGE ( 'NONE', *, *, #6417, .T. ) ;
#14362=VECTOR ( 'NONE', #11077, 1000.000000000000000 ) ;
#14373=EDGE_LOOP ( 'NONE', ( #6745, #20803, #22564, #6890, #1950, #22968, #19152, #11878 ) ) ;
#14381=CARTESIAN_POINT ( 'NONE',  ( -18.35824191589999899, -34.50000000000000000, -142.9407682190000060 ) ) ;
#14391=DIRECTION ( 'NONE',  ( 0.000000000000000000, -1.000000000000000000, -2.765629237170000203E-27 ) ) ;
#14396=AXIS2_PLACEMENT_3D ( 'NONE', #19266, #17250, #8188 ) ;
#14398=CYLINDRICAL_SURFACE ( 'NONE', #10531, 1.000000000000001332 ) ;
#14399=DIRECTION ( 'NONE',  ( 1.000000000000000000, 0.000000000000000000, 0.000000000000000000 ) ) ;
#14414=CARTESIAN_POINT ( 'NONE',  ( 9.683200060760002614, -20.63250393952945316, -148.5552959529999839 ) ) ;
#14417=VECTOR ( 'NONE', #17748, 1000.000000000000000 ) ;
#14433=DIRECTION ( 'NONE',  ( -1.000000000000000000, -3.994014902950000436E-29, 0.000000000000000000 ) ) ;
#14449=ADVANCED_FACE ( 'NONE', ( #9006 ), #5346, .F. ) ;
#14458=DIRECTION ( 'NONE',  ( 1.000000000000000000, 0.000000000000000000, 0.000000000000000000 ) ) ;
#14461=CARTESIAN_POINT ( 'NONE',  ( -21.35824191589999899, -32.00000000000000000, -146.3157682190000060 ) ) ;
#14480=ORIENTED_EDGE ( 'NONE', *, *, #19894, .T. ) ;
#14504=ORIENTED_EDGE ( 'NONE', *, *, #7878, .T. ) ;
#14533=AXIS2_PLACEMENT_3D ( 'NONE', #8097, #12994, #20724 ) ;
#14536=CARTESIAN_POINT ( 'NONE',  ( -34.35824191590000254, -18.00000000000000000, -141.0657682190000060 ) ) ;
#14538=DIRECTION ( 'NONE',  ( 0.000000000000000000, 0.000000000000000000, 1.000000000000000000 ) ) ;
#14548=EDGE_CURVE ( 'NONE', #10902, #9077, #16864, .T. ) ;
#14549=LINE ( 'NONE', #5606, #246 ) ;
#14597=PLANE ( 'NONE',  #6441 ) ;
#14609=CARTESIAN_POINT ( 'NONE',  ( -21.35824191589999899, -31.25000000000000000, -145.5657682190000060 ) ) ;
#14625=ADVANCED_FACE ( 'NONE', ( #4841 ), #7881, .F. ) ;
#14627=DIRECTION ( 'NONE',  ( -2.507771768020000122E-12, 0.000000000000000000, 1.000000000000000000 ) ) ;
#14634=DIRECTION ( 'NONE',  ( -2.423380700840000070E-27, 0.000000000000000000, -1.000000000000000000 ) ) ;
#14636=FACE_OUTER_BOUND ( 'NONE', #13406, .T. ) ;
#14638=ORIENTED_EDGE ( 'NONE', *, *, #20595, .T. ) ;
#14646=ORIENTED_EDGE ( 'NONE', *, *, #393, .F. ) ;
#14657=VECTOR ( 'NONE', #1126, 1000.000000000000000 ) ;
#14679=DIRECTION ( 'NONE',  ( -1.211690350419999855E-27, -2.765629237169980113E-27, 1.000000000000000000 ) ) ;
#14705=FACE_BOUND ( 'NONE', #18744, .T. ) ;
#14735=ORIENTED_EDGE ( 'NONE', *, *, #15241, .T. ) ;
#14756=LINE ( 'NONE', #16891, #2393 ) ;
#14764=ORIENTED_EDGE ( 'NONE', *, *, #2565, .F. ) ;
#14767=AXIS2_PLACEMENT_3D ( 'NONE', #16202, #1589, #5716 ) ;
#14774=CARTESIAN_POINT ( 'NONE',  ( -5.316799939240000938, 3.500000000000000000, -148.5552959529999839 ) ) ;
#14784=EDGE_CURVE ( 'NONE', #21963, #14843, #13265, .T. ) ;
#14787=LINE ( 'NONE', #16682, #6137 ) ;
#14797=VECTOR ( 'NONE', #9596, 1000.000000000000000 ) ;
#14810=CIRCLE ( 'NONE', #19755, 0.7500000000000006661 ) ;
#14816=VERTEX_POINT ( 'NONE', #123 ) ;
#14824=CARTESIAN_POINT ( 'NONE',  ( -22.10824191589999899, -32.00000000000000000, -141.0657682190000060 ) ) ;
#14843=VERTEX_POINT ( 'NONE', #2252 ) ;
#14849=ORIENTED_EDGE ( 'NONE', *, *, #3582, .T. ) ;
#14859=AXIS2_PLACEMENT_3D ( 'NONE', #5084, #19724, #12219 ) ;
#14861=AXIS2_PLACEMENT_3D ( 'NONE', #20275, #11440, #4079 ) ;
#14864=EDGE_CURVE ( 'NONE', #18490, #5042, #7364, .T. ) ;
#14906=FACE_BOUND ( 'NONE', #6944, .T. ) ;
#14907=DIRECTION ( 'NONE',  ( 0.000000000000000000, 1.000000000000000000, 0.000000000000000000 ) ) ;
#14910=LINE ( 'NONE', #22520, #11105 ) ;
#14920=CARTESIAN_POINT ( 'NONE',  ( -21.35824191591069265, -32.00000000000000000, -141.9623572383524959 ) ) ;
#14921=ADVANCED_FACE ( 'NONE', ( #19123 ), #10057, .T. ) ;
#14952=EDGE_LOOP ( 'NONE', ( #355, #15314, #15706, #18843 ) ) ;
#14962=DIRECTION ( 'NONE',  ( 0.000000000000000000, -1.000000000000000000, 0.000000000000000000 ) ) ;
#14969=LINE ( 'NONE', #7702, #21269 ) ;
#15011=AXIS2_PLACEMENT_3D ( 'NONE', #1214, #15818, #8314 ) ;
#15017=ORIENTED_EDGE ( 'NONE', *, *, #3884, .F. ) ;
#15028=EDGE_CURVE ( 'NONE', #8147, #22250, #8751, .T. ) ;
#15035=ORIENTED_EDGE ( 'NONE', *, *, #12973, .F. ) ;
#15043=DIRECTION ( 'NONE',  ( -1.000000000000000000, 0.000000000000000000, 0.000000000000000000 ) ) ;
#15048=DIRECTION ( 'NONE',  ( 3.994014902950000436E-29, -1.000000000000000000, 4.148443855749999753E-27 ) ) ;
#15062=ORIENTED_EDGE ( 'NONE', *, *, #15905, .T. ) ;
#15070=ORIENTED_EDGE ( 'NONE', *, *, #13674, .F. ) ;
#15082=DIRECTION ( 'NONE',  ( -1.211690350419999855E-27, -2.765629237170000203E-27, 1.000000000000000000 ) ) ;
#15090=VERTEX_POINT ( 'NONE', #1402 ) ;
#15094=FACE_BOUND ( 'NONE', #21686, .T. ) ;
#15105=FACE_OUTER_BOUND ( 'NONE', #12582, .T. ) ;
#15110=VECTOR ( 'NONE', #10315, 1000.000000000000000 ) ;
#15123=AXIS2_PLACEMENT_3D ( 'NONE', #14461, #8284, #15558 ) ;
#15132=LINE ( 'NONE', #9641, #20591 ) ;
#15135=ORIENTED_EDGE ( 'NONE', *, *, #11609, .T. ) ;
#15145=EDGE_LOOP ( 'NONE', ( #10511, #19855, #16009, #18285 ) ) ;
#15154=ORIENTED_EDGE ( 'NONE', *, *, #2589, .T. ) ;
#15158=( LENGTH_UNIT ( ) NAMED_UNIT ( * ) SI_UNIT ( .MILLI., .METRE. ) );
#15162=DIRECTION ( 'NONE',  ( -2.507771768019999718E-12, 0.000000000000000000, 1.000000000000000000 ) ) ;
#15176=CARTESIAN_POINT ( 'NONE',  ( 22.68320006080000084, -34.50000000000000000, -149.3052959529999839 ) ) ;
#15183=DIRECTION ( 'NONE',  ( 0.000000000000000000, 0.000000000000000000, 1.000000000000000000 ) ) ;
#15215=EDGE_CURVE ( 'NONE', #4709, #2330, #1880, .T. ) ;
#15241=EDGE_CURVE ( 'NONE', #15634, #18790, #20068, .T. ) ;
#15245=CARTESIAN_POINT ( 'NONE',  ( -5.316799939240000938, 0.9999999999989999111, -148.5552959529999839 ) ) ;
#15256=CARTESIAN_POINT ( 'NONE',  ( 9.810375642909303195, -19.99460661104259884, -148.5552959529999555 ) ) ;
#15257=DIRECTION ( 'NONE',  ( 3.994014902950000436E-29, -1.000000000000000000, 4.148443855749999753E-27 ) ) ;
#15261=ORIENTED_EDGE ( 'NONE', *, *, #9231, .T. ) ;
#15271=AXIS2_PLACEMENT_3D ( 'NONE', #5849, #163, #18585 ) ;
#15285=ORIENTED_EDGE ( 'NONE', *, *, #22728, .T. ) ;
#15292=DIRECTION ( 'NONE',  ( -2.507771768019999718E-12, 0.000000000000000000, 1.000000000000000000 ) ) ;
#15294=ORIENTED_EDGE ( 'NONE', *, *, #7178, .F. ) ;
#15300=CARTESIAN_POINT ( 'NONE',  ( -21.35824191589999899, -4.000000000000000000, -141.0657682190000060 ) ) ;
#15309=CARTESIAN_POINT ( 'NONE',  ( -18.07392865170000107, -1.500000000000000000, -147.3157682190000060 ) ) ;
#15314=ORIENTED_EDGE ( 'NONE', *, *, #16076, .F. ) ;
#15316=CYLINDRICAL_SURFACE ( 'NONE', #11390, 0.7499999999999997780 ) ;
#15341=EDGE_CURVE ( 'NONE', #4100, #22307, #7793, .T. ) ;
#15358=DIRECTION ( 'NONE',  ( 1.000000000000000000, 0.000000000000000000, 0.000000000000000000 ) ) ;
#15359=CARTESIAN_POINT ( 'NONE',  ( -20.60824191589624022, -3.803650459150011542, -146.3157682189980733 ) ) ;
#15364=DIRECTION ( 'NONE',  ( 0.000000000000000000, 1.000000000000000000, 0.000000000000000000 ) ) ;
#15366=DIRECTION ( 'NONE',  ( -1.211690350420779919E-27, -2.765629237169220318E-27, 1.000000000000000000 ) ) ;
#15367=EDGE_CURVE ( 'NONE', #11018, #21963, #16956, .T. ) ;
#15369=EDGE_CURVE ( 'NONE', #14816, #8776, #20737, .T. ) ;
#15371=DIRECTION ( 'NONE',  ( -0.9848077530125619594, 0.000000000000000000, -0.1736481776649230202 ) ) ;
#15403=CARTESIAN_POINT ( 'NONE',  ( -21.35824191589999899, -32.00000000000000000, -146.2257682199999920 ) ) ;
#15408=DIRECTION ( 'NONE',  ( 1.000000000000000000, 0.000000000000000000, 2.507771768020000122E-12 ) ) ;
#15425=CARTESIAN_POINT ( 'NONE',  ( -22.02741209360413777, -3.608510005928772468, -146.3157682189998070 ) ) ;
#15428=ORIENTED_EDGE ( 'NONE', *, *, #2486, .F. ) ;
#15437=EDGE_LOOP ( 'NONE', ( #12954, #3152, #15062, #18683 ) ) ;
#15445=AXIS2_PLACEMENT_3D ( 'NONE', #21071, #1213, #11886 ) ;
#15464=DIRECTION ( 'NONE',  ( 0.000000000000000000, -1.000000000000000000, 0.000000000000000000 ) ) ;
#15467=CARTESIAN_POINT ( 'NONE',  ( -22.10824191589999899, -32.00000000000000000, -145.5657682190000060 ) ) ;
#15470=CARTESIAN_POINT ( 'NONE',  ( 10.68320006080000084, -19.50000000000000000, -150.0552959529999839 ) ) ;
#15484=ORIENTED_EDGE ( 'NONE', *, *, #9650, .T. ) ;
#15515=VERTEX_POINT ( 'NONE', #19575 ) ;
#15516=CARTESIAN_POINT ( 'NONE',  ( -15.46250806109999942, -34.50000000000000000, -147.7289441310000200 ) ) ;
#15531=FACE_OUTER_BOUND ( 'NONE', #4297, .T. ) ;
#15533=ORIENTED_EDGE ( 'NONE', *, *, #8062, .T. ) ;
#15537=DIRECTION ( 'NONE',  ( -3.994014902950000436E-29, 1.000000000000000000, -4.148443855749999753E-27 ) ) ;
#15557=VERTEX_POINT ( 'NONE', #21482 ) ;
#15558=DIRECTION ( 'NONE',  ( 1.000000000000000000, 0.000000000000000000, 2.516505522483685870E-12 ) ) ;
#15560=VERTEX_POINT ( 'NONE', #12409 ) ;
#15581=CARTESIAN_POINT ( 'NONE',  ( -21.35824191589999899, -32.00000000000000000, -144.8157682190000060 ) ) ;
#15585=VERTEX_POINT ( 'NONE', #10153 ) ;
#15634=VERTEX_POINT ( 'NONE', #12186 ) ;
#15636=CARTESIAN_POINT ( 'NONE',  ( -21.35824191591069265, -4.000000000000000000, -141.9623572383524959 ) ) ;
#15646=DIRECTION ( 'NONE',  ( 1.000000000000000000, 0.000000000000000000, 2.516505522483685870E-12 ) ) ;
#15660=AXIS2_PLACEMENT_3D ( 'NONE', #15636, #19320, #10021 ) ;
#15668=CARTESIAN_POINT ( 'NONE',  ( 29.68320006080000084, -24.50000000000000000, -148.5552959529999839 ) ) ;
#15702=DIRECTION ( 'NONE',  ( -2.507771768019999718E-12, -1.592654864209999947E-17, 1.000000000000000000 ) ) ;
#15706=ORIENTED_EDGE ( 'NONE', *, *, #16527, .F. ) ;
#15711=VERTEX_POINT ( 'NONE', #16695 ) ;
#15716=DIRECTION ( 'NONE',  ( 1.000000000000000000, 0.000000000000000000, 2.516505522483685870E-12 ) ) ;
#15739=ORIENTED_EDGE ( 'NONE', *, *, #16819, .F. ) ;
#15745=ORIENTED_EDGE ( 'NONE', *, *, #11707, .T. ) ;
#15758=ORIENTED_EDGE ( 'NONE', *, *, #11609, .F. ) ;
#15759=CARTESIAN_POINT ( 'NONE',  ( -21.35824191589999899, -4.000000000000000000, -144.8157682190000060 ) ) ;
#15783=CARTESIAN_POINT ( 'NONE',  ( 29.68320006080000084, -7.750000000000000000, -150.0552959529999839 ) ) ;
#15796=ORIENTED_EDGE ( 'NONE', *, *, #8750, .F. ) ;
#15803=EDGE_LOOP ( 'NONE', ( #2347, #4368, #9811, #21848 ) ) ;
#15817=DIRECTION ( 'NONE',  ( 1.000000000000000000, 0.000000000000000000, 2.516505522483685870E-12 ) ) ;
#15818=DIRECTION ( 'NONE',  ( 2.507771768019999718E-12, 1.592654864069999939E-17, -1.000000000000000000 ) ) ;
#15824=DIRECTION ( 'NONE',  ( -2.508215857230000030E-12, 0.000000000000000000, 1.000000000000000000 ) ) ;
#15825=LINE ( 'NONE', #6777, #20355 ) ;
#15835=LINE ( 'NONE', #6319, #5847 ) ;
#15844=EDGE_CURVE ( 'NONE', #1, #20629, #4789, .T. ) ;
#15867=DIRECTION ( 'NONE',  ( -2.507771768023035002E-12, -1.592654560756634986E-17, 1.000000000000000000 ) ) ;
#15868=AXIS2_PLACEMENT_3D ( 'NONE', #7131, #13068, #14391 ) ;
#15905=EDGE_CURVE ( 'NONE', #10363, #22236, #6309, .T. ) ;
#15908=DIRECTION ( 'NONE',  ( 0.7071067811865484609, 0.7071067811865466846, 1.776356839400247234E-12 ) ) ;
#15913=DIRECTION ( 'NONE',  ( 3.994014902950000436E-29, -1.000000000000000000, 4.148443855749999753E-27 ) ) ;
#15923=DIRECTION ( 'NONE',  ( 2.507771768019999718E-12, 1.592654864209999947E-17, -1.000000000000000000 ) ) ;
#15927=LINE ( 'NONE', #14381, #6081 ) ;
#15929=EDGE_CURVE ( 'NONE', #3173, #8776, #5862, .T. ) ;
#15933=EDGE_CURVE ( 'NONE', #2396, #22806, #13121, .T. ) ;
#15935=ADVANCED_FACE ( 'NONE', ( #18603 ), #2321, .F. ) ;
#15940=PLANE ( 'NONE',  #15011 ) ;
#15975=EDGE_LOOP ( 'NONE', ( #19617, #20812, #6289, #18447 ) ) ;
#16007=EDGE_LOOP ( 'NONE', ( #13821, #11866, #20226, #3603 ) ) ;
#16009=ORIENTED_EDGE ( 'NONE', *, *, #11345, .F. ) ;
#16031=CARTESIAN_POINT ( 'NONE',  ( -20.60824191589999899, -32.00000000000000000, -145.5657682190000060 ) ) ;
#16050=ORIENTED_EDGE ( 'NONE', *, *, #4008, .T. ) ;
#16057=LINE ( 'NONE', #7248, #8682 ) ;
#16070=DIRECTION ( 'NONE',  ( 1.211690350419999855E-27, 2.765629237170000203E-27, -1.000000000000000000 ) ) ;
#16076=EDGE_CURVE ( 'NONE', #3657, #10194, #1468, .T. ) ;
#16088=FACE_OUTER_BOUND ( 'NONE', #12245, .T. ) ;
#16107=VECTOR ( 'NONE', #15043, 1000.000000000000000 ) ;
#16108=ORIENTED_EDGE ( 'NONE', *, *, #22879, .F. ) ;
#16138=EDGE_LOOP ( 'NONE', ( #15035, #21222, #2020, #22609 ) ) ;
#16168=PLANE ( 'NONE',  #4283 ) ;
#16187=CARTESIAN_POINT ( 'NONE',  ( -22.10824191589999899, -1.500000000000000000, -146.3157682190000060 ) ) ;
#16195=CARTESIAN_POINT ( 'NONE',  ( 9.183200060760000838, -6.500000000000000000, -150.0552959529999839 ) ) ;
#16200=ORIENTED_EDGE ( 'NONE', *, *, #1151, .T. ) ;
#16202=CARTESIAN_POINT ( 'NONE',  ( -5.316799939240000938, 0.9999999999989999111, -150.0552959529999839 ) ) ;
#16204=EDGE_CURVE ( 'NONE', #3040, #6070, #14549, .T. ) ;
#16207=CARTESIAN_POINT ( 'NONE',  ( -18.35824191589999899, -34.50000000000000000, -146.3157682190000060 ) ) ;
#16225=DIRECTION ( 'NONE',  ( -1.000000000000000000, 0.000000000000000000, -2.516505522483685870E-12 ) ) ;
#16231=ORIENTED_EDGE ( 'NONE', *, *, #1613, .T. ) ;
#16232=DIRECTION ( 'NONE',  ( -0.9848077530125620704, 4.409131086918041429E-28, -0.1736481776649230480 ) ) ;
#16243=DIRECTION ( 'NONE',  ( -2.507771768023035002E-12, -1.592654560756634986E-17, 1.000000000000000000 ) ) ;
#16259=VECTOR ( 'NONE', #15824, 1000.000000000000000 ) ;
#16262=VERTEX_POINT ( 'NONE', #13207 ) ;
#16290=ADVANCED_FACE ( 'NONE', ( #4299 ), #4060, .T. ) ;
#16318=CARTESIAN_POINT ( 'NONE',  ( 10.06934556926865376, -21.30022032142531430, -148.5552959529999839 ) ) ;
#16323=AXIS2_PLACEMENT_3D ( 'NONE', #10688, #3327, #17849 ) ;
#16326=VECTOR ( 'NONE', #11487, 1000.000000000000000 ) ;
#16335=CARTESIAN_POINT ( 'NONE',  ( -18.35824191589999899, -13.50000000000000000, -144.8157682190000060 ) ) ;
#16362=AXIS2_PLACEMENT_3D ( 'NONE', #15759, #15867, #23021 ) ;
#16374=ADVANCED_FACE ( 'NONE', ( #8440, #17723, #6892 ), #15940, .T. ) ;
#16375=EDGE_LOOP ( 'NONE', ( #20739, #9519, #3722, #19456 ) ) ;
#16383=EDGE_LOOP ( 'NONE', ( #14191, #5989 ) ) ;
#16412=AXIS2_PLACEMENT_3D ( 'NONE', #9429, #18619, #15162 ) ;
#16417=CARTESIAN_POINT ( 'NONE',  ( -21.35824191589999899, -4.750000000000000000, -146.3157682190075093 ) ) ;
#16433=LINE ( 'NONE', #139, #4963 ) ;
#16441=VERTEX_POINT ( 'NONE', #9980 ) ;
#16446=CARTESIAN_POINT ( 'NONE',  ( -15.90886514219999981, -34.50000000000000000, -148.5657682190000060 ) ) ;
#16450=FACE_OUTER_BOUND ( 'NONE', #16383, .T. ) ;
#16468=CARTESIAN_POINT ( 'NONE',  ( -20.60824191589999899, -32.00000000000000000, -144.8157682190000060 ) ) ;
#16486=CARTESIAN_POINT ( 'NONE',  ( -17.01442029460000072, -34.50000000000000000, -147.5657682190000060 ) ) ;
#16487=EDGE_LOOP ( 'NONE', ( #8878, #10555, #11549, #10606 ) ) ;
#16519=CARTESIAN_POINT ( 'NONE',  ( 18.18320006080000084, 0.4999999999990000776, -149.3052959529999839 ) ) ;
#16527=EDGE_CURVE ( 'NONE', #17890, #3657, #11447, .T. ) ;
#16531=LINE ( 'NONE', #238, #680 ) ;
#16552=FACE_OUTER_BOUND ( 'NONE', #21525, .T. ) ;
#16569=AXIS2_PLACEMENT_3D ( 'NONE', #20392, #9890, #20862 ) ;
#16575=EDGE_CURVE ( 'NONE', #15711, #19530, #10916, .T. ) ;
#16585=PRODUCT_DEFINITION_CONTEXT ( 'detailed design', #8252, 'design' ) ;
#16586=ORIENTED_EDGE ( 'NONE', *, *, #23054, .T. ) ;
#16590=DIRECTION ( 'NONE',  ( 0.000000000000000000, 0.000000000000000000, 1.000000000000000000 ) ) ;
#16601=ADVANCED_FACE ( 'NONE', ( #3804 ), #10560, .F. ) ;
#16662=ORIENTED_EDGE ( 'NONE', *, *, #17386, .F. ) ;
#16679=CARTESIAN_POINT ( 'NONE',  ( 10.42296856120758619, -19.52552649182162270, -148.5552959529999839 ) ) ;
#16682=CARTESIAN_POINT ( 'NONE',  ( 27.18320006080000084, 3.500000000000000000, -149.3052959529999839 ) ) ;
#16687=AXIS2_PLACEMENT_3D ( 'NONE', #10259, #22532, #19433 ) ;
#16695=CARTESIAN_POINT ( 'NONE',  ( -5.316799939240000938, 3.500000000000000000, -150.0552959529999839 ) ) ;
#16707=CIRCLE ( 'NONE', #10994, 0.7500000000000006661 ) ;
#16712=ORIENTED_EDGE ( 'NONE', *, *, #3474, .F. ) ;
#16721=VECTOR ( 'NONE', #20622, 1000.000000000000000 ) ;
#16743=CYLINDRICAL_SURFACE ( 'NONE', #5028, 24.99999999999999645 ) ;
#16755=DIRECTION ( 'NONE',  ( 2.507554887169999917E-12, 0.000000000000000000, -1.000000000000000000 ) ) ;
#16760=DIRECTION ( 'NONE',  ( 2.507554887169999917E-12, 0.000000000000000000, -1.000000000000000000 ) ) ;
#16770=FACE_OUTER_BOUND ( 'NONE', #9933, .T. ) ;
#16773=DIRECTION ( 'NONE',  ( 1.000000000000000000, 0.000000000000000000, 0.000000000000000000 ) ) ;
#16776=DIRECTION ( 'NONE',  ( 1.000000000000000000, 0.000000000000000000, 2.516505522483685870E-12 ) ) ;
#16780=CARTESIAN_POINT ( 'NONE',  ( 11.68320006079999906, -20.50000000000000000, -148.5552959529999839 ) ) ;
#16784=APPLICATION_CONTEXT ( 'automotive_design' ) ;
#16798=CARTESIAN_POINT ( 'NONE',  ( 14.79224200838147318, -1.499999999999999778, -141.9623572382618306 ) ) ;
#16819=EDGE_CURVE ( 'NONE', #6070, #19806, #11957, .T. ) ;
#16860=CARTESIAN_POINT ( 'NONE',  ( -7.816799939239999162, -1.500000000000000000, -150.0552959529999839 ) ) ;
#16864=LINE ( 'NONE', #691, #12489 ) ;
#16891=CARTESIAN_POINT ( 'NONE',  ( 18.18320006080000084, -6.500000000000000000, -149.3052959529999839 ) ) ;
#16904=EDGE_LOOP ( 'NONE', ( #18450, #8052, #20303, #3489 ) ) ;
#16915=CARTESIAN_POINT ( 'NONE',  ( 18.18320006080000084, 0.4999999999990000776, -148.5552959529999839 ) ) ;
#16930=DIRECTION ( 'NONE',  ( 0.000000000000000000, 0.000000000000000000, 1.000000000000000000 ) ) ;
#16936=VERTEX_POINT ( 'NONE', #22293 ) ;
#16944=CARTESIAN_POINT ( 'NONE',  ( 10.68320006080000084, -20.50000000000000000, -150.0552959529999839 ) ) ;
#16956=LINE ( 'NONE', #15176, #6294 ) ;
#16965=ORIENTED_EDGE ( 'NONE', *, *, #3868, .F. ) ;
#16971=LINE ( 'NONE', #11368, #20899 ) ;
#16977=LINE ( 'NONE', #7695, #13304 ) ;
#16979=ORIENTED_EDGE ( 'NONE', *, *, #8364, .F. ) ;
#16984=VECTOR ( 'NONE', #7896, 1000.000000000000000 ) ;
#16995=EDGE_LOOP ( 'NONE', ( #20485, #10232, #22807, #20727 ) ) ;
#17004=CARTESIAN_POINT ( 'NONE',  ( 25.18320006080000084, -34.50000000000000000, -150.0552959529999839 ) ) ;
#17007=VERTEX_POINT ( 'NONE', #13241 ) ;
#17010=CARTESIAN_POINT ( 'NONE',  ( 27.68320006080000084, -32.50000000000000000, -150.0552959529999839 ) ) ;
#17020=AXIS2_PLACEMENT_3D ( 'NONE', #16798, #5730, #18708 ) ;
#17024=VECTOR ( 'NONE', #23175, 1000.000000000000000 ) ;
#17041=ORIENTED_EDGE ( 'NONE', *, *, #17495, .T. ) ;
#17052=AXIS2_PLACEMENT_3D ( 'NONE', #11379, #2133, #2594 ) ;
#17058=LINE ( 'NONE', #22192, #18408 ) ;
#17066=EDGE_CURVE ( 'NONE', #15585, #14843, #2442, .T. ) ;
#17076=VECTOR ( 'NONE', #3577, 1000.000000000000000 ) ;
#17078=EDGE_CURVE ( 'NONE', #6741, #9077, #18839, .T. ) ;
#17082=EDGE_CURVE ( 'NONE', #11018, #15585, #10829, .T. ) ;
#17084=DIRECTION ( 'NONE',  ( 0.000000000000000000, 0.000000000000000000, 1.000000000000000000 ) ) ;
#17085=VERTEX_POINT ( 'NONE', #17405 ) ;
#17097=CARTESIAN_POINT ( 'NONE',  ( 22.68320006080000084, -34.50000000000000000, -150.0552959529999839 ) ) ;
#17102=CARTESIAN_POINT ( 'NONE',  ( -22.10824191589999899, -32.00000000000000000, -150.0657682190000060 ) ) ;
#17109=CARTESIAN_POINT ( 'NONE',  ( 27.18320006080000084, 3.500000000000000000, -150.0552959529999839 ) ) ;
#17111=DIRECTION ( 'NONE',  ( 1.000000000000000000, 0.000000000000000000, 0.000000000000000000 ) ) ;
#17118=VERTEX_POINT ( 'NONE', #10130 ) ;
#17123=DIRECTION ( 'NONE',  ( 2.507771768019999718E-12, 1.592654864069999939E-17, -1.000000000000000000 ) ) ;
#17134=ORIENTED_EDGE ( 'NONE', *, *, #16076, .T. ) ;
#17152=DIRECTION ( 'NONE',  ( 1.000000000000000000, 0.000000000000000000, 2.516505522483685870E-12 ) ) ;
#17158=EDGE_LOOP ( 'NONE', ( #13073, #6213, #19909, #13411 ) ) ;
#17159=CYLINDRICAL_SURFACE ( 'NONE', #12185, 3.500000000000000000 ) ;
#17161=VECTOR ( 'NONE', #21199, 1000.000000000000000 ) ;
#17168=CARTESIAN_POINT ( 'NONE',  ( 0.3832000607639999834, -34.50000000000000000, -149.3052959529999839 ) ) ;
#17177=SHAPE_REPRESENTATION_RELATIONSHIP ( 'NONE' , 'NONE' ,  #23186, #10046 ) ;
#17212=CARTESIAN_POINT ( 'NONE',  ( -21.35824191589999899, -4.750000000000000000, -145.5657682190000060 ) ) ;
#17215=VERTEX_POINT ( 'NONE', #11300 ) ;
#17220=ORIENTED_EDGE ( 'NONE', *, *, #15341, .F. ) ;
#17222=DIRECTION ( 'NONE',  ( 1.000000000000000000, 0.000000000000000000, 0.000000000000000000 ) ) ;
#17240=CARTESIAN_POINT ( 'NONE',  ( -18.35824191589999899, -34.50000000000000000, -146.3157682190000060 ) ) ;
#17250=DIRECTION ( 'NONE',  ( -2.808280234689999718E-18, 1.000000000000000000, 1.592654863659999653E-17 ) ) ;
#17265=CARTESIAN_POINT ( 'NONE',  ( -25.85824191589999899, -13.50000000000000000, -144.8157682190000060 ) ) ;
#17284=LINE ( 'NONE', #10364, #5291 ) ;
#17304=VERTEX_POINT ( 'NONE', #20370 ) ;
#17312=EDGE_LOOP ( 'NONE', ( #7908, #19348, #22569, #9927 ) ) ;
#17323=ORIENTED_EDGE ( 'NONE', *, *, #19945, .F. ) ;
#17327=DIRECTION ( 'NONE',  ( 1.000000000000000000, 0.000000000000000000, 2.504935852220000146E-12 ) ) ;
#17336=DIRECTION ( 'NONE',  ( 1.000000000000000000, 0.000000000000000000, 0.000000000000000000 ) ) ;
#17337=FACE_OUTER_BOUND ( 'NONE', #17158, .T. ) ;
#17359=DIRECTION ( 'NONE',  ( 1.000000000000000000, 0.000000000000000000, 2.516505522483685870E-12 ) ) ;
#17361=DIRECTION ( 'NONE',  ( 1.000000000000000000, 0.000000000000000000, 0.000000000000000000 ) ) ;
#17371=CARTESIAN_POINT ( 'NONE',  ( -21.16189237505000875, -3.249999999999015454, -146.3157682189995512 ) ) ;
#17384=AXIS2_PLACEMENT_3D ( 'NONE', #16446, #12860, #382 ) ;
#17386=EDGE_CURVE ( 'NONE', #19806, #10546, #5114, .T. ) ;
#17395=DIRECTION ( 'NONE',  ( 3.994014902950000436E-29, -1.000000000000000000, 4.148443855749999753E-27 ) ) ;
#17400=AXIS2_PLACEMENT_3D ( 'NONE', #388, #7626, #22863 ) ;
#17405=CARTESIAN_POINT ( 'NONE',  ( -25.35824191590000254, -1.500000000000000000, -144.8157682190000060 ) ) ;
#17409=EDGE_CURVE ( 'NONE', #7389, #1186, #15825, .T. ) ;
#17429=VECTOR ( 'NONE', #5688, 1000.000000000000000 ) ;
#17431=VECTOR ( 'NONE', #17858, 1000.000000000000000 ) ;
#17440=ORIENTED_EDGE ( 'NONE', *, *, #1613, .F. ) ;
#17442=ORIENTED_EDGE ( 'NONE', *, *, #17807, .F. ) ;
#17458=EDGE_CURVE ( 'NONE', #10222, #22806, #1218, .T. ) ;
#17465=VECTOR ( 'NONE', #21631, 1000.000000000000000 ) ;
#17473=CIRCLE ( 'NONE', #10245, 0.7500000000000006661 ) ;
#17479=CIRCLE ( 'NONE', #12917, 3.500000000000000000 ) ;
#17481=ORIENTED_EDGE ( 'NONE', *, *, #17807, .T. ) ;
#17483=CARTESIAN_POINT ( 'NONE',  ( -25.85824191589999899, -34.50000000000000000, -145.5657682190000060 ) ) ;
#17484=ORIENTED_EDGE ( 'NONE', *, *, #6187, .T. ) ;
#17495=EDGE_CURVE ( 'NONE', #17118, #6977, #6897, .T. ) ;
#17506=LINE ( 'NONE', #21207, #9186 ) ;
#17528=CARTESIAN_POINT ( 'NONE',  ( 22.68320006080000084, -24.50000000000000000, -150.0552959529999839 ) ) ;
#17536=ORIENTED_EDGE ( 'NONE', *, *, #11924, .F. ) ;
#17544=VECTOR ( 'NONE', #13818, 1000.000000000000000 ) ;
#17569=EDGE_LOOP ( 'NONE', ( #18, #14292, #21783, #5955 ) ) ;
#17588=CYLINDRICAL_SURFACE ( 'NONE', #1968, 0.7500000000000013323 ) ;
#17618=DIRECTION ( 'NONE',  ( 0.1736481776649230202, 0.000000000000000000, -0.9848077530125619594 ) ) ;
#17625=CYLINDRICAL_SURFACE ( 'NONE', #6888, 10.00000000000000888 ) ;
#17634=ADVANCED_FACE ( 'NONE', ( #22010 ), #7479, .F. ) ;
#17657=EDGE_LOOP ( 'NONE', ( #1254, #2636, #17041, #4052 ) ) ;
#17669=DIRECTION ( 'NONE',  ( 0.000000000000000000, 0.000000000000000000, 1.000000000000000000 ) ) ;
#17673=ORIENTED_EDGE ( 'NONE', *, *, #11166, .F. ) ;
#17690=VERTEX_POINT ( 'NONE', #22354 ) ;
#17698=DIRECTION ( 'NONE',  ( -2.507771768022264771E-12, -1.592655090489709912E-17, 1.000000000000000000 ) ) ;
#17703=FACE_OUTER_BOUND ( 'NONE', #9662, .T. ) ;
#17705=ORIENTED_EDGE ( 'NONE', *, *, #3473, .T. ) ;
#17723=FACE_BOUND ( 'NONE', #1633, .T. ) ;
#17748=DIRECTION ( 'NONE',  ( 0.000000000000000000, 1.000000000000000000, 0.000000000000000000 ) ) ;
#17760=AXIS2_PLACEMENT_3D ( 'NONE', #9305, #17910, #10745 ) ;
#17798=EDGE_CURVE ( 'NONE', #13760, #15090, #704, .T. ) ;
#17806=VECTOR ( 'NONE', #7549, 1000.000000000000227 ) ;
#17807=EDGE_CURVE ( 'NONE', #15585, #2014, #5928, .T. ) ;
#17815=ADVANCED_FACE ( 'NONE', ( #352 ), #2384, .T. ) ;
#17828=AXIS2_PLACEMENT_3D ( 'NONE', #13062, #9704, #7585 ) ;
#17844=DIRECTION ( 'NONE',  ( 2.507771768020000122E-12, -0.000000000000000000, -1.000000000000000000 ) ) ;
#17846=CARTESIAN_POINT ( 'NONE',  ( -20.96728015145808044, -4.669278027980419132, -146.3157682190065145 ) ) ;
#17849=DIRECTION ( 'NONE',  ( 0.7071067811865475727, 0.7071067811865475727, 0.000000000000000000 ) ) ;
#17855=PLANE ( 'NONE',  #13668 ) ;
#17858=DIRECTION ( 'NONE',  ( -1.000000000000000000, 0.000000000000000000, 0.000000000000000000 ) ) ;
#17861=CARTESIAN_POINT ( 'NONE',  ( 0.1832000607640000001, -3.000000000000000000, -150.0552959529999839 ) ) ;
#17886=CARTESIAN_POINT ( 'NONE',  ( -15.61190926919999988, -18.00000000000000000, -146.8816477750000047 ) ) ;
#17888=VECTOR ( 'NONE', #12488, 1000.000000000000000 ) ;
#17890=VERTEX_POINT ( 'NONE', #12098 ) ;
#17910=DIRECTION ( 'NONE',  ( 3.994014902950000436E-29, -1.000000000000000000, 4.148443855749999753E-27 ) ) ;
#17940=CARTESIAN_POINT ( 'NONE',  ( 27.68320006080000084, -34.50000000000000000, -149.3052959529999839 ) ) ;
#17941=ORIENTED_EDGE ( 'NONE', *, *, #3364, .F. ) ;
#17957=CARTESIAN_POINT ( 'NONE',  ( 0.1832000607640000001, -3.000000000000000000, -148.5552959529999839 ) ) ;
#17973=EDGE_CURVE ( 'NONE', #22352, #22041, #20929, .T. ) ;
#17989=CARTESIAN_POINT ( 'NONE',  ( 10.17780667183982501, -21.37282441786776488, -148.5552959529999555 ) ) ;
#17990=ADVANCED_FACE ( 'NONE', ( #19848 ), #3424, .F. ) ;
#18006=CARTESIAN_POINT ( 'NONE',  ( -15.31679993919999916, -34.50000000000000000, -150.0552959529999839 ) ) ;
#18044=LINE ( 'NONE', #10880, #9527 ) ;
#18047=ORIENTED_EDGE ( 'NONE', *, *, #4600, .T. ) ;
#18051=DIRECTION ( 'NONE',  ( 0.7071067811865475727, -0.7071067811865475727, 0.000000000000000000 ) ) ;
#18057=CARTESIAN_POINT ( 'NONE',  ( -14.47770030809999930, -15.50000000000000000, -147.5552959529999839 ) ) ;
#18068=CARTESIAN_POINT ( 'NONE',  ( -22.10824191589999899, -32.00000000000000000, -144.8157682189905984 ) ) ;
#18076=AXIS2_PLACEMENT_3D ( 'NONE', #17528, #23354, #14306 ) ;
#18077=VECTOR ( 'NONE', #3767, 1000.000000000000000 ) ;
#18081=CARTESIAN_POINT ( 'NONE',  ( -20.60824191589999899, -4.099603707729763791, -146.3157682190056619 ) ) ;
#18104=VERTEX_POINT ( 'NONE', #12802 ) ;
#18105=AXIS2_PLACEMENT_3D ( 'NONE', #13583, #8106, #22636 ) ;
#18126=CARTESIAN_POINT ( 'NONE',  ( -25.85824191589999899, -34.50000000000000000, -144.8157682190000060 ) ) ;
#18129=CARTESIAN_POINT ( 'NONE',  ( -17.08912089869999917, -1.500000000000000000, -147.1421200419999877 ) ) ;
#18163=ORIENTED_EDGE ( 'NONE', *, *, #22462, .F. ) ;
#18167=LINE ( 'NONE', #16031, #17465 ) ;
#18169=VECTOR ( 'NONE', #1445, 1000.000000000000000 ) ;
#18188=AXIS2_PLACEMENT_3D ( 'NONE', #17010, #4398, #9856 ) ;
#18198=ORIENTED_EDGE ( 'NONE', *, *, #15933, .F. ) ;
#18207=PLANE ( 'NONE',  #789 ) ;
#18212=EDGE_LOOP ( 'NONE', ( #12019, #18536, #3083, #21260 ) ) ;
#18224=PRODUCT ( 'Deadbolt', 'Deadbolt', '', ( #10624 ) ) ;
#18237=VERTEX_POINT ( 'NONE', #1373 ) ;
#18254=AXIS2_PLACEMENT_3D ( 'NONE', #21652, #6882, #12343 ) ;
#18261=DIRECTION ( 'NONE',  ( 1.561251128379126385E-14, 1.000000000000000000, 0.000000000000000000 ) ) ;
#18285=ORIENTED_EDGE ( 'NONE', *, *, #4982, .T. ) ;
#18328=DIRECTION ( 'NONE',  ( -1.211690350419999855E-27, -2.765629237170000203E-27, 1.000000000000000000 ) ) ;
#18331=CIRCLE ( 'NONE', #2373, 4.000000000000000000 ) ;
#18334=AXIS2_PLACEMENT_3D ( 'NONE', #13083, #6407, #19259 ) ;
#18393=VECTOR ( 'NONE', #20645, 1000.000000000000000 ) ;
#18399=ADVANCED_FACE ( 'NONE', ( #2317 ), #22173, .F. ) ;
#18408=VECTOR ( 'NONE', #5878, 1000.000000000000000 ) ;
#18415=VERTEX_POINT ( 'NONE', #7844 ) ;
#18419=DIRECTION ( 'NONE',  ( 1.000000000000000000, 0.000000000000000000, 0.000000000000000000 ) ) ;
#18424=DIRECTION ( 'NONE',  ( 1.000000000000000000, 0.000000000000000000, 0.000000000000000000 ) ) ;
#18430=FACE_OUTER_BOUND ( 'NONE', #5433, .T. ) ;
#18432=EDGE_LOOP ( 'NONE', ( #22830, #15285, #1047, #1873 ) ) ;
#18445=LINE ( 'NONE', #17004, #11853 ) ;
#18447=ORIENTED_EDGE ( 'NONE', *, *, #978, .F. ) ;
#18450=ORIENTED_EDGE ( 'NONE', *, *, #22462, .T. ) ;
#18464=DIRECTION ( 'NONE',  ( 1.000000000000000000, 0.000000000000000000, 2.516505522483685870E-12 ) ) ;
#18477=FACE_OUTER_BOUND ( 'NONE', #3695, .T. ) ;
#18490=VERTEX_POINT ( 'NONE', #3947 ) ;
#18501=VECTOR ( 'NONE', #19075, 1000.000000000000000 ) ;
#18505=CARTESIAN_POINT ( 'NONE',  ( -21.71608528419999828, -1.500000000000000000, -144.8157682190000060 ) ) ;
#18514=ADVANCED_FACE ( 'NONE', ( #18804 ), #9626, .F. ) ;
#18528=ORIENTED_EDGE ( 'NONE', *, *, #19104, .F. ) ;
#18536=ORIENTED_EDGE ( 'NONE', *, *, #3868, .T. ) ;
#18543=CARTESIAN_POINT ( 'NONE',  ( -21.35824191589999899, -32.75000000000000000, -145.5657682190000060 ) ) ;
#18544=ORIENTED_EDGE ( 'NONE', *, *, #17082, .F. ) ;
#18545=LINE ( 'NONE', #241, #17076 ) ;
#18562=EDGE_CURVE ( 'NONE', #17085, #17118, #21191, .T. ) ;
#18585=DIRECTION ( 'NONE',  ( 0.000000000000000000, 1.592654863519999645E-17, -1.000000000000000000 ) ) ;
#18586=CARTESIAN_POINT ( 'NONE',  ( -22.10824191591069265, -4.000000000000000000, -141.9623572383543717 ) ) ;
#18588=ORIENTED_EDGE ( 'NONE', *, *, #21321, .T. ) ;
#18593=ADVANCED_FACE ( 'NONE', ( #19039 ), #22501, .T. ) ;
#18600=DIRECTION ( 'NONE',  ( 1.211690350419999855E-27, 2.765629237170000203E-27, -1.000000000000000000 ) ) ;
#18603=FACE_OUTER_BOUND ( 'NONE', #4495, .T. ) ;
#18619=DIRECTION ( 'NONE',  ( -1.000000000000000000, -2.808280234649999694E-18, -2.507771768019999718E-12 ) ) ;
#18621=EDGE_CURVE ( 'NONE', #7036, #12734, #2862, .T. ) ;
#18625=CARTESIAN_POINT ( 'NONE',  ( 11.68320006079999906, -20.50000000000000000, -150.0552959529999839 ) ) ;
#18630=AXIS2_PLACEMENT_3D ( 'NONE', #1753, #19831, #10759 ) ;
#18649=DIRECTION ( 'NONE',  ( -2.508215857230000030E-12, 0.000000000000000000, 1.000000000000000000 ) ) ;
#18650=FACE_OUTER_BOUND ( 'NONE', #18432, .T. ) ;
#18662=DIRECTION ( 'NONE',  ( 2.507771768019999718E-12, 1.592654864069999939E-17, -1.000000000000000000 ) ) ;
#18665=AXIS2_PLACEMENT_3D ( 'NONE', #18006, #21463, #14433 ) ;
#18683=ORIENTED_EDGE ( 'NONE', *, *, #13457, .F. ) ;
#18687=EDGE_CURVE ( 'NONE', #4104, #1364, #12712, .T. ) ;
#18691=CARTESIAN_POINT ( 'NONE',  ( 11.29705455228499567, -19.69977967857330725, -148.5552959529999839 ) ) ;
#18705=CIRCLE ( 'NONE', #15660, 0.7500000000000006661 ) ;
#18708=DIRECTION ( 'NONE',  ( -1.000000000000000000, 0.000000000000000000, -2.507771768020000122E-12 ) ) ;
#18712=CARTESIAN_POINT ( 'NONE',  ( 9.683200060759999062, -20.50000000000000000, -148.5552959529999839 ) ) ;
#18726=LINE ( 'NONE', #7869, #11736 ) ;
#18740=LINE ( 'NONE', #9781, #16107 ) ;
#18741=ORIENTED_EDGE ( 'NONE', *, *, #978, .T. ) ;
#18744=EDGE_LOOP ( 'NONE', ( #4715, #14339, #2847, #15533 ) ) ;
#18776=EDGE_CURVE ( 'NONE', #7197, #18490, #7476, .T. ) ;
#18777=CIRCLE ( 'NONE', #22967, 1.000000000000000888 ) ;
#18784=ORIENTED_EDGE ( 'NONE', *, *, #17386, .T. ) ;
#18786=DIRECTION ( 'NONE',  ( 1.000000000000000000, 1.164156988989999824E-17, 2.507771768019999718E-12 ) ) ;
#18790=VERTEX_POINT ( 'NONE', #10559 ) ;
#18794=CARTESIAN_POINT ( 'NONE',  ( 27.18320006080000084, 0.9999999999989999111, -148.5552959529999839 ) ) ;
#18804=FACE_OUTER_BOUND ( 'NONE', #16007, .T. ) ;
#18816=CARTESIAN_POINT ( 'NONE',  ( -34.35824191590000254, -34.50000000000000000, -141.0657682190000060 ) ) ;
#18831=LINE ( 'NONE', #883, #10986 ) ;
#18835=DIRECTION ( 'NONE',  ( -1.000000000000000000, 0.000000000000000000, -2.516505522483685870E-12 ) ) ;
#18837=DIRECTION ( 'NONE',  ( 0.000000000000000000, 0.000000000000000000, 1.000000000000000000 ) ) ;
#18839=LINE ( 'NONE', #2547, #14657 ) ;
#18843=ORIENTED_EDGE ( 'NONE', *, *, #11108, .T. ) ;
#18849=ADVANCED_FACE ( 'NONE', ( #11702 ), #9136, .F. ) ;
#18862=ORIENTED_EDGE ( 'NONE', *, *, #9796, .T. ) ;
#18873=ORIENTED_EDGE ( 'NONE', *, *, #2698, .F. ) ;
#18886=CARTESIAN_POINT ( 'NONE',  ( -18.07392865290000117, -34.50000000000000000, -144.8157682190000060 ) ) ;
#18916=EDGE_CURVE ( 'NONE', #154, #10363, #11262, .T. ) ;
#18917=ORIENTED_EDGE ( 'NONE', *, *, #3473, .F. ) ;
#18918=ORIENTED_EDGE ( 'NONE', *, *, #2486, .T. ) ;
#18921=DIRECTION ( 'NONE',  ( 1.000000000000000000, 3.994014904670000134E-29, -2.423380700840000070E-27 ) ) ;
#18936=DIRECTION ( 'NONE',  ( 0.000000000000000000, 0.000000000000000000, -1.000000000000000000 ) ) ;
#18943=VECTOR ( 'NONE', #14962, 1000.000000000000000 ) ;
#18950=AXIS2_PLACEMENT_3D ( 'NONE', #22965, #4642, #8187 ) ;
#18993=EDGE_CURVE ( 'NONE', #2014, #14816, #23263, .T. ) ;
#19001=DIRECTION ( 'NONE',  ( 0.7071067811865499042, 0.7071067811865451302, 1.776356839400251071E-12 ) ) ;
#19028=DIRECTION ( 'NONE',  ( 1.000000000000000000, 0.000000000000000000, 2.516505522483685870E-12 ) ) ;
#19037=VECTOR ( 'NONE', #21583, 1000.000000000000000 ) ;
#19039=FACE_OUTER_BOUND ( 'NONE', #5404, .T. ) ;
#19059=CARTESIAN_POINT ( 'NONE',  ( 27.68320006080000084, -34.50000000000000000, -148.5552959529999839 ) ) ;
#19064=VERTEX_POINT ( 'NONE', #4704 ) ;
#19070=DIRECTION ( 'NONE',  ( 0.000000000000000000, 0.000000000000000000, 1.000000000000000000 ) ) ;
#19074=DIRECTION ( 'NONE',  ( -2.507771768020000122E-12, -0.000000000000000000, 1.000000000000000000 ) ) ;
#19075=DIRECTION ( 'NONE',  ( 0.000000000000000000, 0.000000000000000000, 1.000000000000000000 ) ) ;
#19085=ORIENTED_EDGE ( 'NONE', *, *, #437, .F. ) ;
#19089=VECTOR ( 'NONE', #8515, 1000.000000000000000 ) ;
#19104=EDGE_CURVE ( 'NONE', #7140, #5042, #4056, .T. ) ;
#19118=DIRECTION ( 'NONE',  ( 0.000000000000000000, 1.000000000000000000, 0.000000000000000000 ) ) ;
#19123=FACE_OUTER_BOUND ( 'NONE', #12286, .T. ) ;
#19139=VECTOR ( 'NONE', #9561, 1000.000000000000000 ) ;
#19143=PLANE ( 'NONE',  #161 ) ;
#19150=DIRECTION ( 'NONE',  ( 2.510584333019999972E-12, 0.000000000000000000, -1.000000000000000000 ) ) ;
#19152=ORIENTED_EDGE ( 'NONE', *, *, #4898, .F. ) ;
#19165=CARTESIAN_POINT ( 'NONE',  ( -17.08912089869999917, -18.00000000000000000, -147.1421200419999877 ) ) ;
#19183=EDGE_LOOP ( 'NONE', ( #4384, #17442, #6583, #11524 ) ) ;
#19203=CYLINDRICAL_SURFACE ( 'NONE', #16362, 0.7500000000000013323 ) ;
#19215=EDGE_LOOP ( 'NONE', ( #3952, #21328, #12673, #2378 ) ) ;
#19218=EDGE_LOOP ( 'NONE', ( #6104, #1059, #19518, #3249 ) ) ;
#19221=DIRECTION ( 'NONE',  ( 1.000000000000000000, 0.000000000000000000, 0.000000000000000000 ) ) ;
#19240=ADVANCED_FACE ( 'NONE', ( #12535 ), #19816, .T. ) ;
#19242=CARTESIAN_POINT ( 'NONE',  ( -14.47770030809999930, -34.50000000000000000, -148.5552959529999839 ) ) ;
#19259=DIRECTION ( 'NONE',  ( -0.7071067811865481278, -0.7071067811865469066, -1.776356839400246426E-12 ) ) ;
#19264=CARTESIAN_POINT ( 'NONE',  ( 24.68320006080000084, -16.50000000000000000, -150.0552959529999839 ) ) ;
#19266=CARTESIAN_POINT ( 'NONE',  ( -9.766576661180000229, -34.50000000000000000, -145.5657682190000060 ) ) ;
#19282=CARTESIAN_POINT ( 'NONE',  ( -21.35824191589999899, -32.00000000000000000, -146.2257682199999920 ) ) ;
#19320=DIRECTION ( 'NONE',  ( -2.507771768020000122E-12, -0.000000000000000000, 1.000000000000000000 ) ) ;
#19321=CARTESIAN_POINT ( 'NONE',  ( 11.68320006079999906, -20.50000000000000000, -148.5552959529999839 ) ) ;
#19327=ORIENTED_EDGE ( 'NONE', *, *, #23052, .F. ) ;
#19338=VECTOR ( 'NONE', #12469, 1000.000000000000000 ) ;
#19348=ORIENTED_EDGE ( 'NONE', *, *, #2565, .T. ) ;
#19357=PRESENTATION_STYLE_ASSIGNMENT (( #3067 ) ) ;
#19408=LINE ( 'NONE', #8906, #3828 ) ;
#19409=DIRECTION ( 'NONE',  ( -1.211690350420779919E-27, -2.765629237169220318E-27, 1.000000000000000000 ) ) ;
#19433=DIRECTION ( 'NONE',  ( 0.000000000000000000, -4.148443855749999753E-27, -1.000000000000000000 ) ) ;
#19450=CARTESIAN_POINT ( 'NONE',  ( 10.94499944859915530, -21.50000000000000355, -148.5552959529999839 ) ) ;
#19453=CARTESIAN_POINT ( 'NONE',  ( -15.90886514219999981, -1.500000000000000000, -148.5657682190000060 ) ) ;
#19456=ORIENTED_EDGE ( 'NONE', *, *, #14108, .F. ) ;
#19469=AXIS2_PLACEMENT_3D ( 'NONE', #9717, #18786, #13658 ) ;
#19492=DIRECTION ( 'NONE',  ( -2.507771768019999718E-12, -1.592654864209999947E-17, 1.000000000000000000 ) ) ;
#19495=ORIENTED_EDGE ( 'NONE', *, *, #11116, .T. ) ;
#19511=DIRECTION ( 'NONE',  ( 2.507771768020000122E-12, -0.000000000000000000, -1.000000000000000000 ) ) ;
#19518=ORIENTED_EDGE ( 'NONE', *, *, #11166, .T. ) ;
#19530=VERTEX_POINT ( 'NONE', #14774 ) ;
#19570=EDGE_CURVE ( 'NONE', #10546, #15560, #3953, .T. ) ;
#19575=CARTESIAN_POINT ( 'NONE',  ( 10.68320006080000084, -21.50000000000000000, -150.0552959529999839 ) ) ;
#19603=AXIS2_PLACEMENT_3D ( 'NONE', #8016, #11823, #22664 ) ;
#19605=LINE ( 'NONE', #17940, #12947 ) ;
#19609=ORIENTED_EDGE ( 'NONE', *, *, #21019, .F. ) ;
#19611=DIRECTION ( 'NONE',  ( 1.000000000000000000, 0.000000000000000000, 0.000000000000000000 ) ) ;
#19617=ORIENTED_EDGE ( 'NONE', *, *, #3801, .T. ) ;
#19622=VERTEX_POINT ( 'NONE', #15470 ) ;
#19648=DIRECTION ( 'NONE',  ( 0.1736481776649230202, 0.000000000000000000, -0.9848077530125619594 ) ) ;
#19662=ORIENTED_EDGE ( 'NONE', *, *, #2649, .T. ) ;
#19681=EDGE_CURVE ( 'NONE', #2494, #5644, #13923, .T. ) ;
#19684=DIRECTION ( 'NONE',  ( 2.507771768019999718E-12, 1.592654864209999947E-17, -1.000000000000000000 ) ) ;
#19700=LINE ( 'NONE', #10872, #402 ) ;
#19711=DIRECTION ( 'NONE',  ( 1.000000000000000000, 0.000000000000000000, 0.000000000000000000 ) ) ;
#19724=DIRECTION ( 'NONE',  ( 2.507771768020000122E-12, -0.000000000000000000, -1.000000000000000000 ) ) ;
#19739=ORIENTED_EDGE ( 'NONE', *, *, #5055, .F. ) ;
#19743=VERTEX_POINT ( 'NONE', #10690 ) ;
#19755=AXIS2_PLACEMENT_3D ( 'NONE', #21543, #3571, #10563 ) ;
#19762=CIRCLE ( 'NONE', #23167, 0.7500000000000006661 ) ;
#19764=FACE_OUTER_BOUND ( 'NONE', #20059, .T. ) ;
#19766=VECTOR ( 'NONE', #1060, 1000.000000000000000 ) ;
#19806=VERTEX_POINT ( 'NONE', #21900 ) ;
#19815=FACE_OUTER_BOUND ( 'NONE', #23398, .T. ) ;
#19816=PLANE ( 'NONE',  #17760 ) ;
#19822=EDGE_LOOP ( 'NONE', ( #17220, #19609 ) ) ;
#19827=CARTESIAN_POINT ( 'NONE',  ( -25.35824191590000254, -34.50000000000000000, -145.5657682199999954 ) ) ;
#19829=ORIENTED_EDGE ( 'NONE', *, *, #4008, .F. ) ;
#19831=DIRECTION ( 'NONE',  ( -2.507771768019999718E-12, -1.592654864069999939E-17, 1.000000000000000000 ) ) ;
#19848=FACE_OUTER_BOUND ( 'NONE', #7063, .T. ) ;
#19849=ORIENTED_EDGE ( 'NONE', *, *, #10863, .F. ) ;
#19853=EDGE_CURVE ( 'NONE', #4100, #18237, #2492, .T. ) ;
#19855=ORIENTED_EDGE ( 'NONE', *, *, #6850, .F. ) ;
#19857=ORIENTED_EDGE ( 'NONE', *, *, #7201, .F. ) ;
#19859=FACE_OUTER_BOUND ( 'NONE', #16904, .T. ) ;
#19874=CARTESIAN_POINT ( 'NONE',  ( 14.79224200838147318, -1.499999999999999778, -141.9623572382618306 ) ) ;
#19888=DIRECTION ( 'NONE',  ( 1.000000000000000000, 0.000000000000000000, 0.000000000000000000 ) ) ;
#19894=EDGE_CURVE ( 'NONE', #1194, #963, #16531, .T. ) ;
#19908=DIRECTION ( 'NONE',  ( -0.7071067811865499042, 0.7071067811865451302, -1.776356839400251071E-12 ) ) ;
#19909=ORIENTED_EDGE ( 'NONE', *, *, #15341, .T. ) ;
#19917=EDGE_CURVE ( 'NONE', #9077, #8849, #12445, .T. ) ;
#19927=CARTESIAN_POINT ( 'NONE',  ( -20.60824191589999899, -32.00000000000000000, -146.2257682199999920 ) ) ;
#19945=EDGE_CURVE ( 'NONE', #14843, #14816, #6277, .T. ) ;
#19947=ORIENTED_EDGE ( 'NONE', *, *, #4952, .F. ) ;
#19963=( GEOMETRIC_REPRESENTATION_CONTEXT ( 3 ) GLOBAL_UNCERTAINTY_ASSIGNED_CONTEXT ( ( #8258 ) ) GLOBAL_UNIT_ASSIGNED_CONTEXT ( ( #2820, #8039, #9817 ) ) REPRESENTATION_CONTEXT ( 'NONE', 'WORKASPACE' ) );
#19977=AXIS2_PLACEMENT_3D ( 'NONE', #13013, #21843, #14458 ) ;
#19991=DIRECTION ( 'NONE',  ( 1.000000000000000000, 3.994014904670000134E-29, -2.423380700840000070E-27 ) ) ;
#19993=DIRECTION ( 'NONE',  ( -1.211690350419999855E-27, -2.765629237170000203E-27, 1.000000000000000000 ) ) ;
#20009=EDGE_CURVE ( 'NONE', #21283, #7036, #3079, .T. ) ;
#20027=EDGE_CURVE ( 'NONE', #2330, #22041, #5445, .T. ) ;
#20038=FACE_OUTER_BOUND ( 'NONE', #9598, .T. ) ;
#20042=AXIS2_PLACEMENT_3D ( 'NONE', #3511, #16243, #10623 ) ;
#20044=B_SPLINE_CURVE_WITH_KNOTS ( 'NONE', 3,
 ( #733, #17371, #4527, #8088, #15359, #7970 ),
 .UNSPECIFIED., .F., .F.,
 ( 4, 2, 4 ),
 ( 0.000000000000000000, 0.5000000000000000000, 1.000000000000000000 ),
 .UNSPECIFIED. ) ;
#20053=ORIENTED_EDGE ( 'NONE', *, *, #17458, .F. ) ;
#20059=EDGE_LOOP ( 'NONE', ( #19662, #22384, #11392, #3897 ) ) ;
#20068=LINE ( 'NONE', #9443, #18077 ) ;
#20075=EDGE_LOOP ( 'NONE', ( #18047, #8694, #15294, #23367 ) ) ;
#20084=EDGE_LOOP ( 'NONE', ( #11476, #8897, #2093, #10572 ) ) ;
#20089=CARTESIAN_POINT ( 'NONE',  ( -9.766576661180000229, -18.00000000000000000, -145.5657682190000060 ) ) ;
#20090=PLANE ( 'NONE',  #9798 ) ;
#20104=FACE_BOUND ( 'NONE', #8670, .T. ) ;
#20116=ORIENTED_EDGE ( 'NONE', *, *, #21618, .F. ) ;
#20117=CARTESIAN_POINT ( 'NONE',  ( -15.31679993919999916, -18.00000000000000000, -148.5552959529999839 ) ) ;
#20122=DIRECTION ( 'NONE',  ( -3.994014902950000436E-29, 1.000000000000000000, -4.148443855749999753E-27 ) ) ;
#20125=ORIENTED_EDGE ( 'NONE', *, *, #22728, .F. ) ;
#20142=CARTESIAN_POINT ( 'NONE',  ( -21.35824191589999899, -4.000000000000000000, -150.0657682190000060 ) ) ;
#20166=CARTESIAN_POINT ( 'NONE',  ( -17.08912089869999917, -34.50000000000000000, -147.1421200419999877 ) ) ;
#20178=UNCERTAINTY_MEASURE_WITH_UNIT (LENGTH_MEASURE( 1.000000000000000082E-05 ), #15158, 'distance_accuracy_value', 'NONE');
#20180=FILL_AREA_STYLE_COLOUR ( '', #483 ) ;
#20203=AXIS2_PLACEMENT_3D ( 'NONE', #20117, #487, #3933 ) ;
#20226=ORIENTED_EDGE ( 'NONE', *, *, #21618, .T. ) ;
#20227=CARTESIAN_POINT ( 'NONE',  ( -22.10824191589999899, -4.000000000000000000, -146.2257682199999920 ) ) ;
#20241=AXIS2_PLACEMENT_3D ( 'NONE', #21883, #10905, #3315 ) ;
#20263=CYLINDRICAL_SURFACE ( 'NONE', #17400, 1.000000000000001332 ) ;
#20266=CARTESIAN_POINT ( 'NONE',  ( 10.55069612126581724, -19.50000000000000355, -148.5552959529999839 ) ) ;
#20275=CARTESIAN_POINT ( 'NONE',  ( -14.47770030809999930, -34.50000000000000000, -147.5552959529999839 ) ) ;
#20285=FACE_OUTER_BOUND ( 'NONE', #22332, .T. ) ;
#20288=DIRECTION ( 'NONE',  ( -0.7071067811865499042, -0.7071067811865451302, -1.776356839400251071E-12 ) ) ;
#20303=ORIENTED_EDGE ( 'NONE', *, *, #11064, .T. ) ;
#20308=CARTESIAN_POINT ( 'NONE',  ( -22.10824191589999899, -1.500000000000000000, -144.8157682190000060 ) ) ;
#20319=ADVANCED_FACE ( 'NONE', ( #15531 ), #6365, .F. ) ;
#20346=EDGE_CURVE ( 'NONE', #576, #12024, #4354, .T. ) ;
#20347=DIRECTION ( 'NONE',  ( 1.000000000000000000, 0.000000000000000000, 2.516505522483685870E-12 ) ) ;
#20351=DIRECTION ( 'NONE',  ( 1.211690350419999855E-27, 2.765629237170000203E-27, -1.000000000000000000 ) ) ;
#20355=VECTOR ( 'NONE', #20962, 1000.000000000000000 ) ;
#20357=CARTESIAN_POINT ( 'NONE',  ( -22.02741209360413777, -4.391489994071226199, -146.3157682190016828 ) ) ;
#20370=CARTESIAN_POINT ( 'NONE',  ( -15.61190926919999988, -1.500000000000000000, -146.8816477750000047 ) ) ;
#20373=DIRECTION ( 'NONE',  ( 2.507771768019999718E-12, 1.592654864209999947E-17, -1.000000000000000000 ) ) ;
#20380=LINE ( 'NONE', #8099, #9273 ) ;
#20385=AXIS2_PLACEMENT_3D ( 'NONE', #22411, #6106, #4910 ) ;
#20389=CARTESIAN_POINT ( 'NONE',  ( 0.3832000607639999834, -34.50000000000000000, -148.5552959529999839 ) ) ;
#20392=CARTESIAN_POINT ( 'NONE',  ( -21.35824191589999899, -4.000000000000000000, -150.0657682190000060 ) ) ;
#20402=ORIENTED_EDGE ( 'NONE', *, *, #3025, .F. ) ;
#20478=ORIENTED_EDGE ( 'NONE', *, *, #3251, .T. ) ;
#20483=CARTESIAN_POINT ( 'NONE',  ( 29.68320006080000084, -32.50000000000000000, -150.0552959529999839 ) ) ;
#20485=ORIENTED_EDGE ( 'NONE', *, *, #15929, .F. ) ;
#20515=AXIS2_PLACEMENT_3D ( 'NONE', #1762, #23171, #18051 ) ;
#20521=AXIS2_PLACEMENT_3D ( 'NONE', #2959, #13788, #4738 ) ;
#20550=CIRCLE ( 'NONE', #12573, 1.000000000000000888 ) ;
#20554=CARTESIAN_POINT ( 'NONE',  ( -21.35824191589999899, -32.00000000000000000, -144.8157682190000060 ) ) ;
#20587=CARTESIAN_POINT ( 'NONE',  ( -21.35824191589999899, -32.00000000000000000, -144.8157682190000060 ) ) ;
#20589=CARTESIAN_POINT ( 'NONE',  ( -22.10824191589999899, -4.000000000000000000, -146.3157682190000060 ) ) ;
#20590=CLOSED_SHELL ( 'NONE', ( #12248, #8531, #21538, #17990, #22621, #5157, #7293, #8031, #7892, #6231, #21910, #8437, #3935, #16601, #3150, #11660, #11484, #18593, #13483, #13235, #14921, #16290, #8077, #8789, #5855, #1765, #4701, #19240, #11035, #18399, #12001, #11849, #11407, #12455, #1407, #8495, #15935, #6303, #6343, #23300, #640, #7052, #17815, #7776, #7316, #18849, #13327, #13418, #7648, #16374, #14336, #172, #14449, #12714, #18514, #827, #22906, #23223, #11343, #6183, #17634, #10706, #256 ) ) ;
#20591=VECTOR ( 'NONE', #4072, 1000.000000000000000 ) ;
#20594=CARTESIAN_POINT ( 'NONE',  ( 11.48351823926500437, -19.88604765140169661, -148.5552959529999839 ) ) ;
#20595=EDGE_CURVE ( 'NONE', #9931, #19743, #2872, .T. ) ;
#20598=VERTEX_POINT ( 'NONE', #11773 ) ;
#20622=DIRECTION ( 'NONE',  ( 2.507554887169999917E-12, 0.000000000000000000, -1.000000000000000000 ) ) ;
#20629=VERTEX_POINT ( 'NONE', #10347 ) ;
#20632=CARTESIAN_POINT ( 'NONE',  ( -34.35824191590000254, -34.50000000000000000, -150.0657682190000060 ) ) ;
#20645=DIRECTION ( 'NONE',  ( -1.000000000000000000, 0.000000000000000000, 0.000000000000000000 ) ) ;
#20671=CARTESIAN_POINT ( 'NONE',  ( -21.71608528380000180, -34.50000000000000000, -146.3157682190000060 ) ) ;
#20678=DIRECTION ( 'NONE',  ( 0.9848077530125619594, 0.000000000000000000, 0.1736481776649230202 ) ) ;
#20706=ORIENTED_EDGE ( 'NONE', *, *, #21019, .T. ) ;
#20710=DIRECTION ( 'NONE',  ( -2.423380700840000070E-27, 0.000000000000000000, -1.000000000000000000 ) ) ;
#20723=MECHANICAL_DESIGN_GEOMETRIC_PRESENTATION_REPRESENTATION('',(#209),#19963);
#20724=DIRECTION ( 'NONE',  ( 1.000000000000000000, 0.000000000000000000, 2.516505522483685870E-12 ) ) ;
#20727=ORIENTED_EDGE ( 'NONE', *, *, #15369, .T. ) ;
#20737=CIRCLE ( 'NONE', #19603, 10.00000000000000000 ) ;
#20739=ORIENTED_EDGE ( 'NONE', *, *, #2514, .F. ) ;
#20743=EDGE_CURVE ( 'NONE', #1513, #1364, #136, .T. ) ;
#20745=FACE_OUTER_BOUND ( 'NONE', #12586, .T. ) ;
#20756=VECTOR ( 'NONE', #11864, 1000.000000000000000 ) ;
#20758=DIRECTION ( 'NONE',  ( -2.507771768019999718E-12, -1.592654864069999939E-17, 1.000000000000000000 ) ) ;
#20773=DIRECTION ( 'NONE',  ( 0.9848077530125619594, 0.000000000000000000, 0.1736481776649230202 ) ) ;
#20774=ORIENTED_EDGE ( 'NONE', *, *, #393, .T. ) ;
#20776=ORIENTED_EDGE ( 'NONE', *, *, #6768, .T. ) ;
#20778=ORIENTED_EDGE ( 'NONE', *, *, #12190, .T. ) ;
#20787=VECTOR ( 'NONE', #3450, 1000.000000000000000 ) ;
#20803=ORIENTED_EDGE ( 'NONE', *, *, #13478, .T. ) ;
#20812=ORIENTED_EDGE ( 'NONE', *, *, #7785, .T. ) ;
#20819=CARTESIAN_POINT ( 'NONE',  ( -21.35824191589999899, -31.25000000000000000, -146.3157682190075093 ) ) ;
#20828=DIRECTION ( 'NONE',  ( -1.000000000000000000, 0.000000000000000000, 0.000000000000000000 ) ) ;
#20840=VERTEX_POINT ( 'NONE', #9022 ) ;
#20862=DIRECTION ( 'NONE',  ( 1.000000000000000000, 0.000000000000000000, 2.516505522483685870E-12 ) ) ;
#20882=CARTESIAN_POINT ( 'NONE',  ( -25.85824191589999899, -34.50000000000000000, -146.3157682190000060 ) ) ;
#20886=FACE_OUTER_BOUND ( 'NONE', #14952, .T. ) ;
#20899=VECTOR ( 'NONE', #18649, 1000.000000000000000 ) ;
#20909=ORIENTED_EDGE ( 'NONE', *, *, #3703, .T. ) ;
#20916=AXIS2_PLACEMENT_3D ( 'NONE', #9786, #15048, #11691 ) ;
#20929=LINE ( 'NONE', #5087, #20756 ) ;
#20933=FACE_BOUND ( 'NONE', #13333, .T. ) ;
#20952=CIRCLE ( 'NONE', #14859, 0.7500000000000006661 ) ;
#20954=ORIENTED_EDGE ( 'NONE', *, *, #3107, .F. ) ;
#20962=DIRECTION ( 'NONE',  ( 2.506794771760000178E-12, 0.000000000000000000, -1.000000000000000000 ) ) ;
#21000=AXIS2_PLACEMENT_3D ( 'NONE', #20587, #4050, #491 ) ;
#21003=CARTESIAN_POINT ( 'NONE',  ( 0.1832000607640000001, -6.500000000000000000, -148.5552959529999839 ) ) ;
#21019=EDGE_CURVE ( 'NONE', #22307, #4100, #3375, .T. ) ;
#21027=ORIENTED_EDGE ( 'NONE', *, *, #2558, .T. ) ;
#21071=CARTESIAN_POINT ( 'NONE',  ( -7.816799939239999162, 0.9999999999989999111, -150.0552959529999839 ) ) ;
#21127=CARTESIAN_POINT ( 'NONE',  ( -20.60824191589999899, -32.00000000000000000, -141.0657682190000060 ) ) ;
#21141=ORIENTED_EDGE ( 'NONE', *, *, #17973, .T. ) ;
#21191=LINE ( 'NONE', #1083, #14296 ) ;
#21199=DIRECTION ( 'NONE',  ( 2.507554887169999917E-12, 0.000000000000000000, -1.000000000000000000 ) ) ;
#21207=CARTESIAN_POINT ( 'NONE',  ( -16.20111387579999729, -1.500000000000000000, -147.8591802640000026 ) ) ;
#21208=CARTESIAN_POINT ( 'NONE',  ( 9.183200060760000838, -6.500000000000000000, -148.5552959529999839 ) ) ;
#21218=AXIS2_PLACEMENT_3D ( 'NONE', #4215, #22072, #2444 ) ;
#21222=ORIENTED_EDGE ( 'NONE', *, *, #1963, .T. ) ;
#21260=ORIENTED_EDGE ( 'NONE', *, *, #13911, .F. ) ;
#21263=CARTESIAN_POINT ( 'NONE',  ( -20.60824191589999899, -4.000000000000000000, -144.8157682190000060 ) ) ;
#21269=VECTOR ( 'NONE', #20678, 1000.000000000000227 ) ;
#21283=VERTEX_POINT ( 'NONE', #22445 ) ;
#21295=CIRCLE ( 'NONE', #3817, 1.000000000000000888 ) ;
#21298=EDGE_CURVE ( 'NONE', #18790, #17304, #13246, .T. ) ;
#21321=EDGE_CURVE ( 'NONE', #15557, #12276, #17284, .T. ) ;
#21328=ORIENTED_EDGE ( 'NONE', *, *, #13026, .T. ) ;
#21333=B_SPLINE_CURVE_WITH_KNOTS ( 'NONE', 3,
 ( #10022, #19450, #14089, #12051, #10490, #19321 ),
 .UNSPECIFIED., .F., .F.,
 ( 4, 2, 4 ),
 ( 0.000000000000000000, 0.5000000000000000000, 1.000000000000000000 ),
 .UNSPECIFIED. ) ;
#21350=ORIENTED_EDGE ( 'NONE', *, *, #14864, .T. ) ;
#21358=ORIENTED_EDGE ( 'NONE', *, *, #15933, .T. ) ;
#21432=CARTESIAN_POINT ( 'NONE',  ( 10.68320006080000084, -20.50000000000000000, -148.5552959529999839 ) ) ;
#21433=CARTESIAN_POINT ( 'NONE',  ( -21.71608528380000180, -1.500000000000000000, -144.8157682190000060 ) ) ;
#21434=CARTESIAN_POINT ( 'NONE',  ( 9.183200060760000838, -6.500000000000000000, -148.5552959529999839 ) ) ;
#21435=ORIENTED_EDGE ( 'NONE', *, *, #22890, .F. ) ;
#21441=CYLINDRICAL_SURFACE ( 'NONE', #863, 0.7500000000000006661 ) ;
#21443=EDGE_LOOP ( 'NONE', ( #1576, #21027, #1072, #17536 ) ) ;
#21447=ORIENTED_EDGE ( 'NONE', *, *, #23485, .T. ) ;
#21461=AXIS2_PLACEMENT_3D ( 'NONE', #3587, #23222, #7029 ) ;
#21463=DIRECTION ( 'NONE',  ( 3.994014902950000436E-29, -1.000000000000000000, 4.148443855749999753E-27 ) ) ;
#21482=CARTESIAN_POINT ( 'NONE',  ( 29.68320006080000084, -24.50000000000000000, -150.0552959529999839 ) ) ;
#21494=VECTOR ( 'NONE', #4562, 1000.000000000000000 ) ;
#21516=CARTESIAN_POINT ( 'NONE',  ( -14.47770030809999930, -15.50000000000000000, -148.5552959529999839 ) ) ;
#21522=DIRECTION ( 'NONE',  ( -2.508215857230000030E-12, 0.000000000000000000, 1.000000000000000000 ) ) ;
#21525=EDGE_LOOP ( 'NONE', ( #15739, #7659, #892, #11436 ) ) ;
#21528=DIRECTION ( 'NONE',  ( -2.507771768020000122E-12, 0.000000000000000000, 1.000000000000000000 ) ) ;
#21532=DIRECTION ( 'NONE',  ( 2.506794771760000178E-12, 0.000000000000000000, -1.000000000000000000 ) ) ;
#21538=ADVANCED_FACE ( 'NONE', ( #20745 ), #4560, .F. ) ;
#21543=CARTESIAN_POINT ( 'NONE',  ( -21.35824191589999899, -4.000000000000000000, -144.8157682190000060 ) ) ;
#21547=DIRECTION ( 'NONE',  ( -2.507771768019999718E-12, -1.592654864069999939E-17, 1.000000000000000000 ) ) ;
#21567=ORIENTED_EDGE ( 'NONE', *, *, #22668, .F. ) ;
#21583=DIRECTION ( 'NONE',  ( -1.000000000000000000, 0.000000000000000000, -2.506439500389999993E-12 ) ) ;
#21617=CARTESIAN_POINT ( 'NONE',  ( -25.35824191589811960, -1.500000000000000000, -146.3157682190081630 ) ) ;
#21618=EDGE_CURVE ( 'NONE', #22236, #10363, #10605, .T. ) ;
#21626=CARTESIAN_POINT ( 'NONE',  ( -15.46250806109999942, -1.500000000000000000, -147.7289441310000200 ) ) ;
#21631=DIRECTION ( 'NONE',  ( -2.508215857230000030E-12, 0.000000000000000000, 1.000000000000000000 ) ) ;
#21652=CARTESIAN_POINT ( 'NONE',  ( 0.3832000607639999834, -24.50000000000000000, -150.0552959529999839 ) ) ;
#21654=CARTESIAN_POINT ( 'NONE',  ( -18.35824191589999899, -1.500000000000000000, -150.0657682190000060 ) ) ;
#21673=CARTESIAN_POINT ( 'NONE',  ( 10.68320006080000084, -21.50000000000000000, -148.5552959529999839 ) ) ;
#21674=FACE_OUTER_BOUND ( 'NONE', #17312, .T. ) ;
#21686=EDGE_LOOP ( 'NONE', ( #5155, #13368, #12263, #8828 ) ) ;
#21689=ORIENTED_EDGE ( 'NONE', *, *, #9796, .F. ) ;
#21698=ORIENTED_EDGE ( 'NONE', *, *, #2698, .T. ) ;
#21703=LINE ( 'NONE', #17886, #13737 ) ;
#21715=DIRECTION ( 'NONE',  ( 1.000000000000000000, 0.000000000000000000, 2.516505522483685870E-12 ) ) ;
#21745=ORIENTED_EDGE ( 'NONE', *, *, #676, .T. ) ;
#21770=EDGE_CURVE ( 'NONE', #9931, #3657, #20044, .T. ) ;
#21783=ORIENTED_EDGE ( 'NONE', *, *, #5060, .T. ) ;
#21836=EDGE_CURVE ( 'NONE', #6188, #10194, #14810, .T. ) ;
#21843=DIRECTION ( 'NONE',  ( -3.994014902950000436E-29, 1.000000000000000000, -4.148443855749999753E-27 ) ) ;
#21848=ORIENTED_EDGE ( 'NONE', *, *, #1837, .F. ) ;
#21849=FILL_AREA_STYLE ('',( #20180 ) ) ;
#21862=ORIENTED_EDGE ( 'NONE', *, *, #4333, .T. ) ;
#21872=DIRECTION ( 'NONE',  ( 0.6427876096872939815, 0.000000000000000000, 0.7660444431183448533 ) ) ;
#21883=CARTESIAN_POINT ( 'NONE',  ( 27.18320006080000084, 3.500000000000000000, -150.0552959529999839 ) ) ;
#21897=FACE_OUTER_BOUND ( 'NONE', #5329, .T. ) ;
#21900=CARTESIAN_POINT ( 'NONE',  ( -15.61190926919999988, -34.50000000000000000, -146.8816477750000047 ) ) ;
#21904=DIRECTION ( 'NONE',  ( -2.507771768019999718E-12, -1.592654864069999939E-17, 1.000000000000000000 ) ) ;
#21910=ADVANCED_FACE ( 'NONE', ( #1326 ), #23087, .F. ) ;
#21911=CARTESIAN_POINT ( 'NONE',  ( -22.10824191589999899, -32.00000000000000000, -146.2257682199999920 ) ) ;
#21934=CIRCLE ( 'NONE', #2934, 0.7500000000000006661 ) ;
#21960=FACE_OUTER_BOUND ( 'NONE', #4178, .T. ) ;
#21963=VERTEX_POINT ( 'NONE', #472 ) ;
#21996=EDGE_LOOP ( 'NONE', ( #3783, #20774, #17484, #8860 ) ) ;
#21999=AXIS2_PLACEMENT_3D ( 'NONE', #11094, #18600, #9193 ) ;
#22008=VERTEX_POINT ( 'NONE', #17109 ) ;
#22009=CARTESIAN_POINT ( 'NONE',  ( -9.766576661180000229, -1.500000000000000000, -145.5657682190000060 ) ) ;
#22010=FACE_OUTER_BOUND ( 'NONE', #8043, .T. ) ;
#22011=CIRCLE ( 'NONE', #17828, 0.7500000000000006661 ) ;
#22023=CARTESIAN_POINT ( 'NONE',  ( -21.35824191589999899, -4.750000000000000000, -146.3157682190075093 ) ) ;
#22028=ORIENTED_EDGE ( 'NONE', *, *, #1259, .F. ) ;
#22041=VERTEX_POINT ( 'NONE', #19242 ) ;
#22047=EDGE_CURVE ( 'NONE', #5391, #10427, #9910, .T. ) ;
#22050=FACE_OUTER_BOUND ( 'NONE', #27, .T. ) ;
#22061=CARTESIAN_POINT ( 'NONE',  ( -34.35824191590000254, -1.500000000000000000, -141.0657682190000060 ) ) ;
#22066=ADVANCED_FACE ( 'NONE', ( #8285 ), #9954, .F. ) ;
#22072=DIRECTION ( 'NONE',  ( 2.507771768019999718E-12, 1.592654864069999939E-17, -1.000000000000000000 ) ) ;
#22075=ORIENTED_EDGE ( 'NONE', *, *, #15369, .F. ) ;
#22110=CARTESIAN_POINT ( 'NONE',  ( 29.68320006080000084, -28.50000000000000000, -148.5552959529999839 ) ) ;
#22116=CIRCLE ( 'NONE', #1617, 0.7500000000000006661 ) ;
#22126=EDGE_LOOP ( 'NONE', ( #6532, #21350, #16231, #11531 ) ) ;
#22132=CARTESIAN_POINT ( 'NONE',  ( -21.35824191589999899, -4.000000000000000000, -141.0657682190000060 ) ) ;
#22140=DIRECTION ( 'NONE',  ( -0.1736481776649230202, 0.000000000000000000, 0.9848077530125619594 ) ) ;
#22152=DIRECTION ( 'NONE',  ( 0.000000000000000000, 0.000000000000000000, 1.000000000000000000 ) ) ;
#22154=ORIENTED_EDGE ( 'NONE', *, *, #17798, .T. ) ;
#22157=PLANE ( 'NONE',  #17020 ) ;
#22163=PLANE ( 'NONE',  #15271 ) ;
#22173=PLANE ( 'NONE',  #18105 ) ;
#22175=CYLINDRICAL_SURFACE ( 'NONE', #12151, 4.000000000000000000 ) ;
#22176=ORIENTED_EDGE ( 'NONE', *, *, #23054, .F. ) ;
#22188=( NAMED_UNIT ( * ) PLANE_ANGLE_UNIT ( ) SI_UNIT ( $, .RADIAN. ) );
#22192=CARTESIAN_POINT ( 'NONE',  ( 29.68320006080000084, -16.50000000000000000, -149.3052959529999839 ) ) ;
#22193=EDGE_CURVE ( 'NONE', #11758, #154, #20952, .T. ) ;
#22202=EDGE_CURVE ( 'NONE', #16936, #3124, #19605, .T. ) ;
#22236=VERTEX_POINT ( 'NONE', #3543 ) ;
#22250=VERTEX_POINT ( 'NONE', #14248 ) ;
#22263=DIRECTION ( 'NONE',  ( -2.508215857230000030E-12, 0.000000000000000000, 1.000000000000000000 ) ) ;
#22291=DIRECTION ( 'NONE',  ( 1.000000000000000000, 0.000000000000000000, 0.000000000000000000 ) ) ;
#22293=CARTESIAN_POINT ( 'NONE',  ( 27.68320006080000084, -34.50000000000000000, -150.0552959529999839 ) ) ;
#22307=VERTEX_POINT ( 'NONE', #3188 ) ;
#22310=ADVANCED_FACE ( 'NONE', ( #3077 ), #17588, .F. ) ;
#22314=DIRECTION ( 'NONE',  ( 0.000000000000000000, 1.592654863519999645E-17, -1.000000000000000000 ) ) ;
#22332=EDGE_LOOP ( 'NONE', ( #18198, #7571, #2882, #5349 ) ) ;
#22334=LINE ( 'NONE', #2588, #22793 ) ;
#22352=VERTEX_POINT ( 'NONE', #23528 ) ;
#22354=CARTESIAN_POINT ( 'NONE',  ( -18.35824191589999899, -34.50000000000000000, -141.0657682190000060 ) ) ;
#22355=ORIENTED_EDGE ( 'NONE', *, *, #18562, .F. ) ;
#22364=CIRCLE ( 'NONE', #14767, 2.500000000000000000 ) ;
#22384=ORIENTED_EDGE ( 'NONE', *, *, #2957, .F. ) ;
#22411=CARTESIAN_POINT ( 'NONE',  ( -17.23482902069999767, -18.00000000000000000, -146.3157682190000060 ) ) ;
#22427=CARTESIAN_POINT ( 'NONE',  ( 18.18320006080000084, -6.500000000000000000, -150.0552959529999839 ) ) ;
#22445=CARTESIAN_POINT ( 'NONE',  ( 29.68320006080000084, 0.9999999999989999111, -148.5552959529999839 ) ) ;
#22448=CARTESIAN_POINT ( 'NONE',  ( 19.68320006079999729, -24.50000000000000000, -148.5552959529999839 ) ) ;
#22461=LINE ( 'NONE', #13172, #17429 ) ;
#22462=EDGE_CURVE ( 'NONE', #22008, #15711, #5782, .T. ) ;
#22468=CIRCLE ( 'NONE', #443, 3.500000000000000000 ) ;
#22473=CARTESIAN_POINT ( 'NONE',  ( 11.53320006080000049, -24.50000000000000000, -150.0552959529999839 ) ) ;
#22483=EDGE_CURVE ( 'NONE', #10783, #17304, #796, .T. ) ;
#22501=PLANE ( 'NONE',  #15445 ) ;
#22515=CYLINDRICAL_SURFACE ( 'NONE', #14533, 0.7500000000000006661 ) ;
#22520=CARTESIAN_POINT ( 'NONE',  ( 29.68320006080000084, -32.50000000000000000, -149.3052959529999839 ) ) ;
#22525=AXIS2_PLACEMENT_3D ( 'NONE', #1043, #6617, #6150 ) ;
#22528=EDGE_LOOP ( 'NONE', ( #22075, #17323, #3212, #14504, #21745, #15017, #11525, #5150, #7425, #4096, #18862, #9508, #2671, #9805, #18918, #2122, #9097 ) ) ;
#22532=DIRECTION ( 'NONE',  ( -3.994014902950000436E-29, 1.000000000000000000, -4.148443855749999753E-27 ) ) ;
#22564=ORIENTED_EDGE ( 'NONE', *, *, #2129, .T. ) ;
#22569=ORIENTED_EDGE ( 'NONE', *, *, #18621, .T. ) ;
#22576=SURFACE_STYLE_FILL_AREA ( #10301 ) ;
#22589=EDGE_CURVE ( 'NONE', #15515, #1861, #9574, .T. ) ;
#22591=DIRECTION ( 'NONE',  ( -1.211690350419999855E-27, -2.765629237170000203E-27, 1.000000000000000000 ) ) ;
#22605=CARTESIAN_POINT ( 'NONE',  ( 11.68320006080000262, -20.36749606047844807, -148.5552959529999839 ) ) ;
#22606=CYLINDRICAL_SURFACE ( 'NONE', #18188, 2.000000000000001776 ) ;
#22609=ORIENTED_EDGE ( 'NONE', *, *, #20743, .F. ) ;
#22621=ADVANCED_FACE ( 'NONE', ( #14196 ), #3719, .T. ) ;
#22636=DIRECTION ( 'NONE',  ( 0.000000000000000000, -4.148443855749999753E-27, -1.000000000000000000 ) ) ;
#22639=CARTESIAN_POINT ( 'NONE',  ( 9.683200060759999062, -20.50000000000000000, -150.0552959529999839 ) ) ;
#22661=CARTESIAN_POINT ( 'NONE',  ( 9.183200060760000838, 0.4999999999990000776, -150.0552959529999839 ) ) ;
#22664=DIRECTION ( 'NONE',  ( 1.000000000000000000, 0.000000000000000000, 0.000000000000000000 ) ) ;
#22668=EDGE_CURVE ( 'NONE', #19806, #17304, #21703, .T. ) ;
#22671=ADVANCED_FACE ( 'NONE', ( #1604 ), #23357, .F. ) ;
#22702=EDGE_LOOP ( 'NONE', ( #9575, #22867, #13308, #5458 ) ) ;
#22728=EDGE_CURVE ( 'NONE', #13760, #20840, #10680, .T. ) ;
#22741=DIRECTION ( 'NONE',  ( 3.994014902950000436E-29, -1.000000000000000000, 4.148443855749999753E-27 ) ) ;
#22766=EDGE_LOOP ( 'NONE', ( #9967, #21358, #13347, #22355 ) ) ;
#22793=VECTOR ( 'NONE', #13513, 1000.000000000000000 ) ;
#22802=ORIENTED_EDGE ( 'NONE', *, *, #4600, .F. ) ;
#22806=VERTEX_POINT ( 'NONE', #973 ) ;
#22807=ORIENTED_EDGE ( 'NONE', *, *, #18993, .T. ) ;
#22830=ORIENTED_EDGE ( 'NONE', *, *, #17798, .F. ) ;
#22843=DIRECTION ( 'NONE',  ( 1.000000000000000000, 0.000000000000000000, 2.516505522483685870E-12 ) ) ;
#22858=ORIENTED_EDGE ( 'NONE', *, *, #7497, .T. ) ;
#22863=DIRECTION ( 'NONE',  ( -0.7071067811865475727, -0.7071067811865475727, 0.000000000000000000 ) ) ;
#22865=DIRECTION ( 'NONE',  ( -2.508215857230000030E-12, 0.000000000000000000, 1.000000000000000000 ) ) ;
#22867=ORIENTED_EDGE ( 'NONE', *, *, #13674, .T. ) ;
#22879=EDGE_CURVE ( 'NONE', #8780, #10783, #11897, .T. ) ;
#22890=EDGE_CURVE ( 'NONE', #6977, #7870, #22978, .T. ) ;
#22901=CARTESIAN_POINT ( 'NONE',  ( -25.85824191589999899, -34.50000000000000000, -144.8157682190000060 ) ) ;
#22906=ADVANCED_FACE ( 'NONE', ( #4770 ), #12017, .F. ) ;
#22917=EDGE_CURVE ( 'NONE', #7197, #7140, #6663, .T. ) ;
#22935=EDGE_CURVE ( 'NONE', #16936, #7230, #6514, .T. ) ;
#22938=PRODUCT_DEFINITION_FORMATION_WITH_SPECIFIED_SOURCE ( 'ANY', '', #18224, .NOT_KNOWN. ) ;
#22951=ORIENTED_EDGE ( 'NONE', *, *, #11865, .T. ) ;
#22965=CARTESIAN_POINT ( 'NONE',  ( -34.35824191590000254, -34.50000000000000000, -141.0657682190000060 ) ) ;
#22967=AXIS2_PLACEMENT_3D ( 'NONE', #16944, #11811, #9430 ) ;
#22968=ORIENTED_EDGE ( 'NONE', *, *, #2016, .F. ) ;
#22978=LINE ( 'NONE', #17265, #17544 ) ;
#22979=EDGE_CURVE ( 'NONE', #9016, #12276, #12722, .T. ) ;
#22985=DIRECTION ( 'NONE',  ( 2.507771768019999718E-12, 1.592654864209999947E-17, -1.000000000000000000 ) ) ;
#22996=CARTESIAN_POINT ( 'NONE',  ( -20.60824191589999899, -4.000000000000000000, -145.5657682190000060 ) ) ;
#23004=CARTESIAN_POINT ( 'NONE',  ( -16.35051508389999597, -1.500000000000000000, -147.0118839079999873 ) ) ;
#23021=DIRECTION ( 'NONE',  ( -0.7071067811865484609, 0.7071067811865466846, -1.776356839400247234E-12 ) ) ;
#23030=ORIENTED_EDGE ( 'NONE', *, *, #5060, .F. ) ;
#23052=EDGE_CURVE ( 'NONE', #22250, #18790, #23211, .T. ) ;
#23054=EDGE_CURVE ( 'NONE', #17215, #15634, #3459, .T. ) ;
#23083=VERTEX_POINT ( 'NONE', #1801 ) ;
#23084=CARTESIAN_POINT ( 'NONE',  ( -21.35824191589185972, -32.00000000000000000, -149.4708568729758724 ) ) ;
#23087=CYLINDRICAL_SURFACE ( 'NONE', #16323, 1.000000000000001332 ) ;
#23135=ORIENTED_EDGE ( 'NONE', *, *, #4898, .T. ) ;
#23167=AXIS2_PLACEMENT_3D ( 'NONE', #10325, #15923, #10203 ) ;
#23170=AXIS2_PLACEMENT_3D ( 'NONE', #3094, #19511, #17359 ) ;
#23171=DIRECTION ( 'NONE',  ( -1.211690350420779919E-27, -2.765629237169220318E-27, 1.000000000000000000 ) ) ;
#23175=DIRECTION ( 'NONE',  ( 0.000000000000000000, -1.000000000000000000, 0.000000000000000000 ) ) ;
#23183=EDGE_LOOP ( 'NONE', ( #18741, #16979, #1534, #10419 ) ) ;
#23186=SHAPE_REPRESENTATION ( 'Deadbolt', ( #5025 ), #5047 ) ;
#23191=AXIS2_PLACEMENT_3D ( 'NONE', #15581, #15702, #22843 ) ;
#23211=LINE ( 'NONE', #21433, #12214 ) ;
#23222=DIRECTION ( 'NONE',  ( 2.507771768020000122E-12, -0.000000000000000000, -1.000000000000000000 ) ) ;
#23223=ADVANCED_FACE ( 'NONE', ( #14636 ), #9608, .F. ) ;
#23243=LINE ( 'NONE', #46, #19037 ) ;
#23246=ORIENTED_EDGE ( 'NONE', *, *, #3592, .T. ) ;
#23263=LINE ( 'NONE', #3048, #5581 ) ;
#23272=ORIENTED_EDGE ( 'NONE', *, *, #8750, .T. ) ;
#23280=ORIENTED_EDGE ( 'NONE', *, *, #15844, .F. ) ;
#23300=ADVANCED_FACE ( 'NONE', ( #1061 ), #7941, .F. ) ;
#23309=EDGE_LOOP ( 'NONE', ( #13510, #15758, #6494, #5740 ) ) ;
#23310=CARTESIAN_POINT ( 'NONE',  ( -25.85824191589999899, -1.500000000000000000, -146.3157682190000060 ) ) ;
#23326=DIRECTION ( 'NONE',  ( 1.000000000000000000, 0.000000000000000000, 0.000000000000000000 ) ) ;
#23354=DIRECTION ( 'NONE',  ( 1.211690350419999855E-27, 2.765629237170000203E-27, -1.000000000000000000 ) ) ;
#23357=CYLINDRICAL_SURFACE ( 'NONE', #8778, 0.7499999999999997780 ) ;
#23365=DIRECTION ( 'NONE',  ( -2.507771768019999718E-12, -1.592654864069999939E-17, 1.000000000000000000 ) ) ;
#23367=ORIENTED_EDGE ( 'NONE', *, *, #16575, .F. ) ;
#23384=ORIENTED_EDGE ( 'NONE', *, *, #531, .T. ) ;
#23398=EDGE_LOOP ( 'NONE', ( #6425, #16050, #14638, #5023 ) ) ;
#23404=VECTOR ( 'NONE', #9368, 1000.000000000000000 ) ;
#23425=DIRECTION ( 'NONE',  ( 1.000000000000000000, 0.000000000000000000, 0.000000000000000000 ) ) ;
#23435=DIRECTION ( 'NONE',  ( -1.000000000000000000, 0.000000000000000000, -2.507771768020000122E-12 ) ) ;
#23440=DIRECTION ( 'NONE',  ( 1.000000000000000000, 0.000000000000000000, 2.516505522483685870E-12 ) ) ;
#23458=DIRECTION ( 'NONE',  ( 0.000000000000000000, -1.000000000000000000, -1.592654864069999939E-17 ) ) ;
#23462=DIRECTION ( 'NONE',  ( 1.000000000000000000, 0.000000000000000000, 2.504935852220000146E-12 ) ) ;
#23475=DIRECTION ( 'NONE',  ( 3.994014902950000436E-29, -1.000000000000000000, 4.148443855749999753E-27 ) ) ;
#23485=EDGE_CURVE ( 'NONE', #12734, #9016, #18331, .T. ) ;
#23510=ORIENTED_EDGE ( 'NONE', *, *, #1837, .T. ) ;
#23525=VERTEX_POINT ( 'NONE', #2928 ) ;
#23528=CARTESIAN_POINT ( 'NONE',  ( -14.47770030809999930, -34.50000000000000000, -150.0552959529999839 ) ) ;
ENDSEC;
END-ISO-10303-21;
